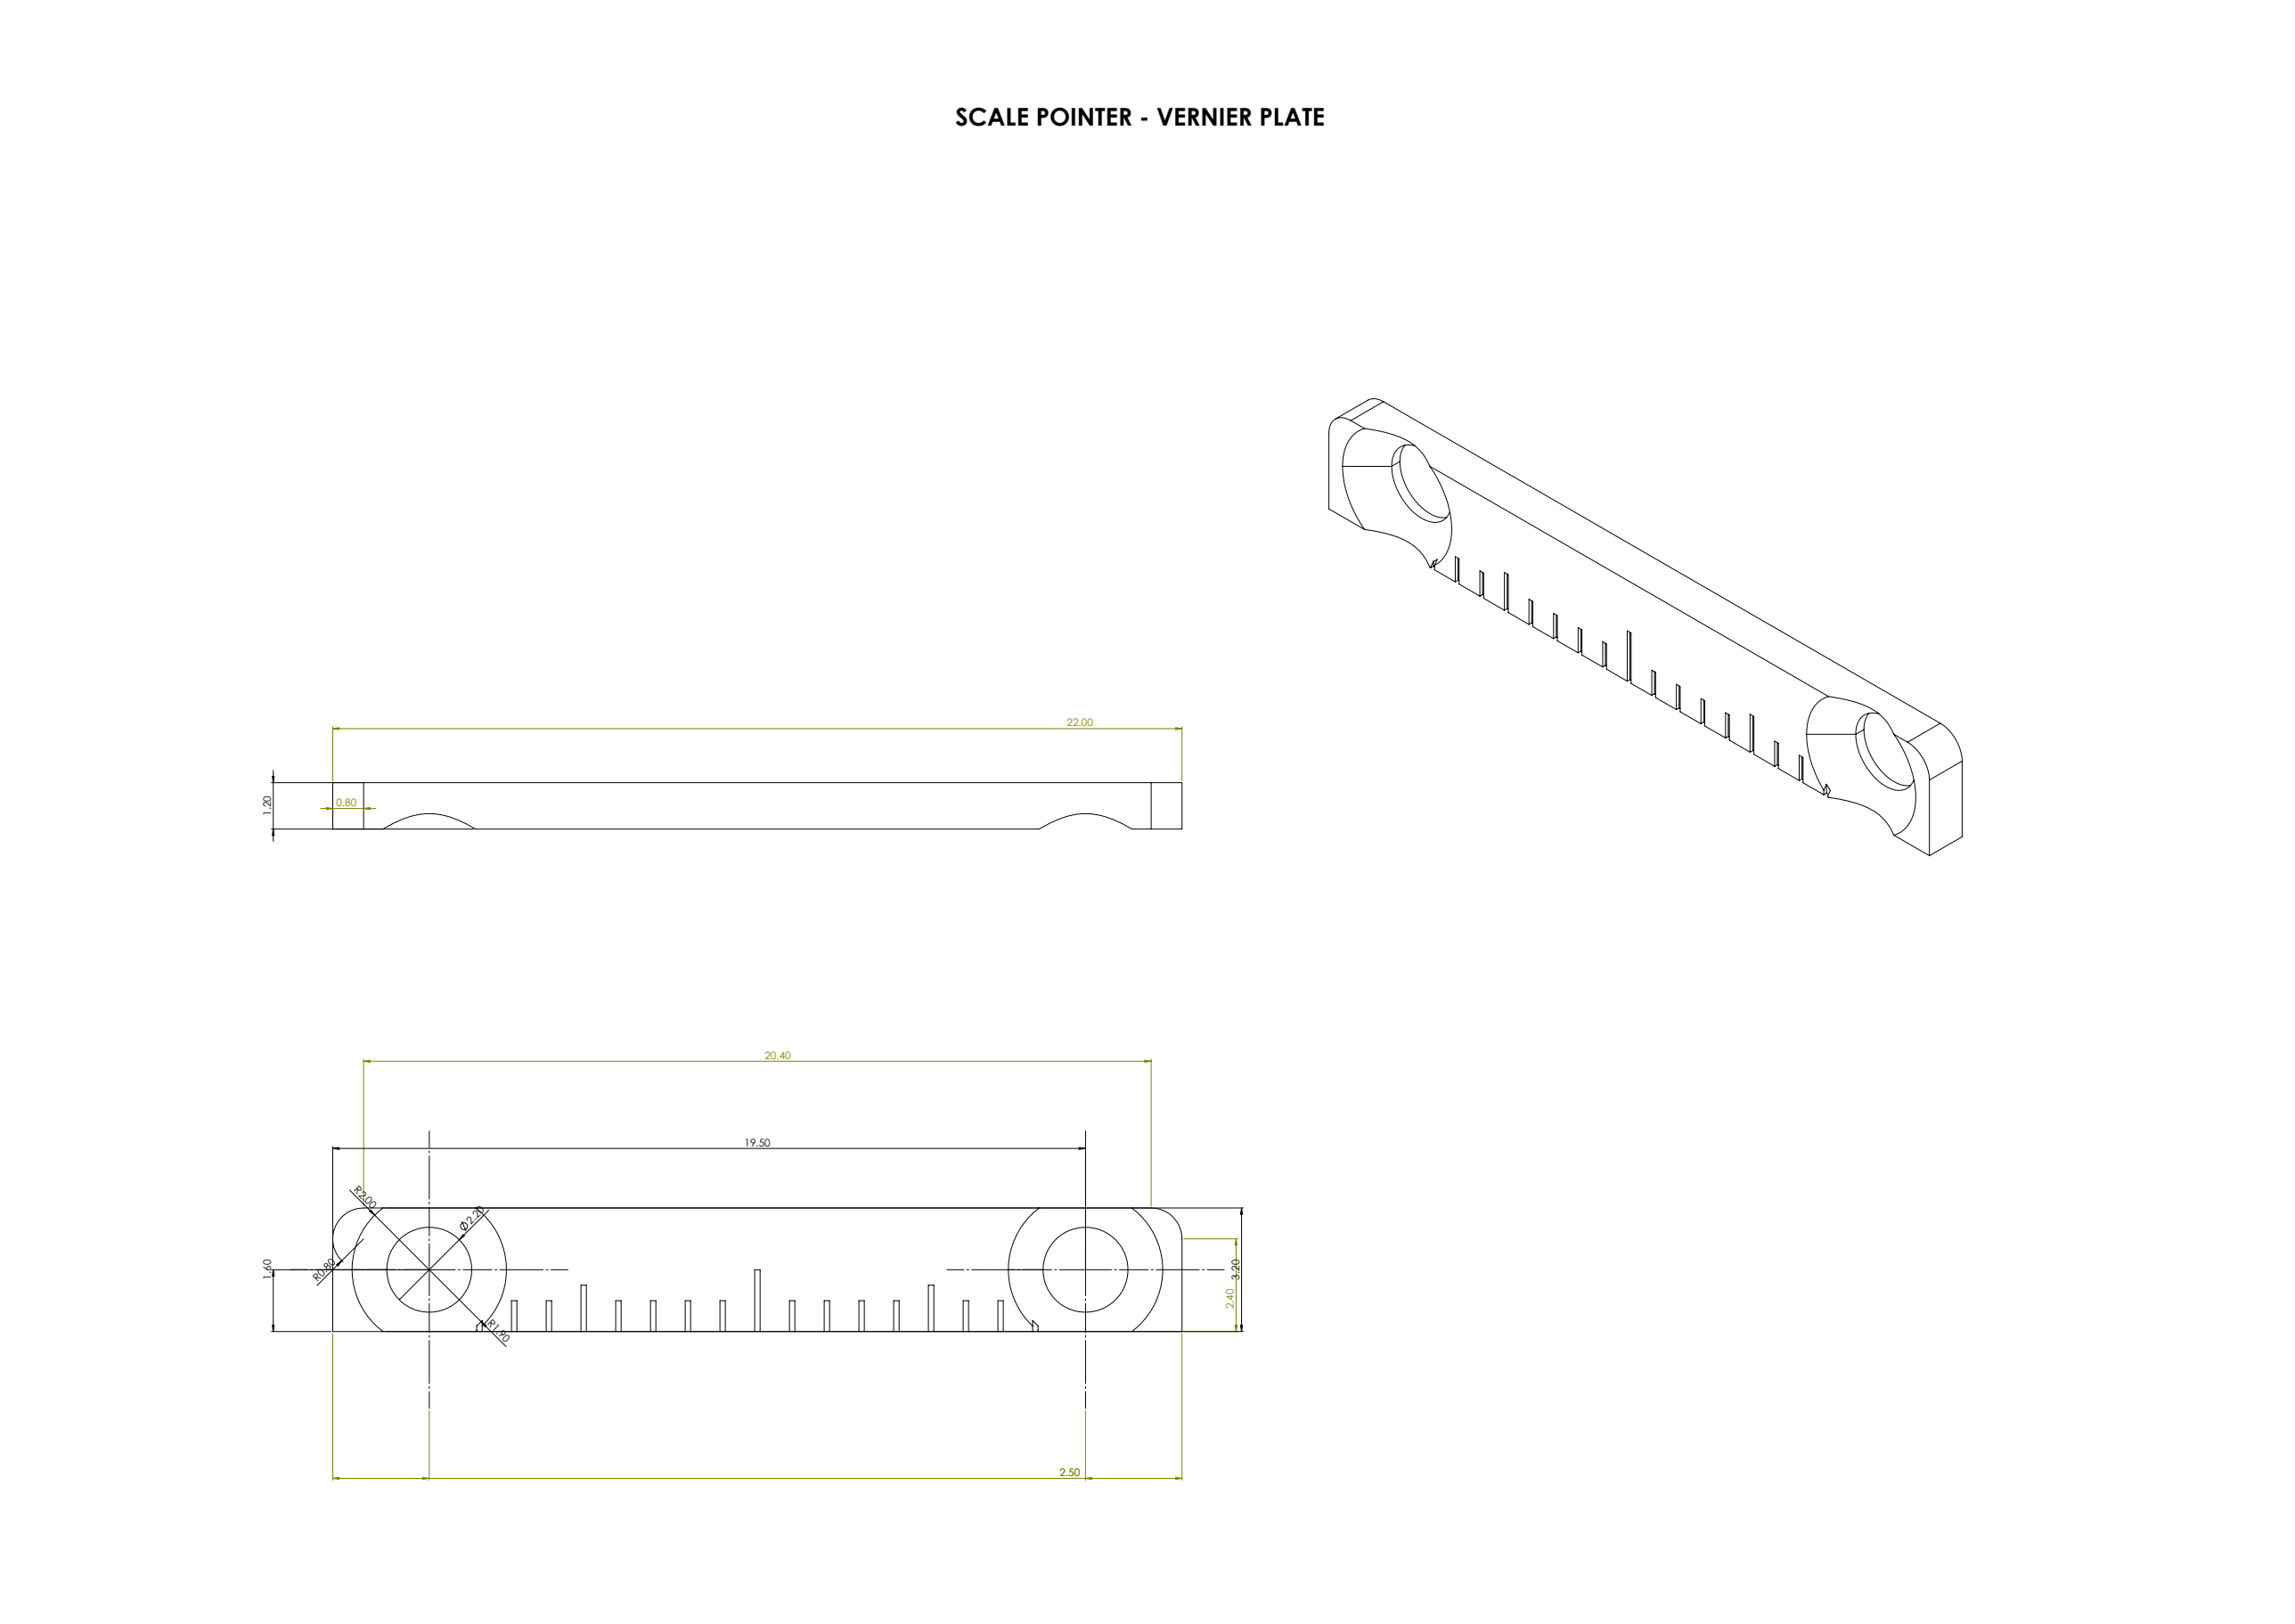
ISO-10303-21;
HEADER;
/* Generated by software containing ST-Developer
 * from STEP Tools, Inc. (www.steptools.com) 
 */

FILE_DESCRIPTION(
/* description */ (''),
/* implementation_level */ '2;1');

FILE_NAME(
/* name */ 'Scale Pointer - Vernier Plate.step',
/* time_stamp */ '2026-10-05T09:57:53+05:00',
/* author */ (''),
/* organization */ (''),
/* preprocessor_version */ 'ST-DEVELOPER v20.2',
/* originating_system */ 'Autodesk Translation Framework v15.15.0.0',
/* authorisation */ '');

FILE_SCHEMA (('AUTOMOTIVE_DESIGN { 1 0 10303 214 3 1 1 }'));
ENDSEC;

DATA;
#10=MECHANICAL_DESIGN_GEOMETRIC_PRESENTATION_REPRESENTATION('',(#560),#113984);
#371=(
BOUNDED_CURVE()
B_SPLINE_CURVE(2,(#102311,#102312,#102313),.UNSPECIFIED.,.F.,.F.)
B_SPLINE_CURVE_WITH_KNOTS((3,3),(0.,0.017254918292991),.UNSPECIFIED.)
CURVE()
GEOMETRIC_REPRESENTATION_ITEM()
RATIONAL_B_SPLINE_CURVE((1.,1.000650607336,1.))
REPRESENTATION_ITEM('')
);
#372=(
BOUNDED_CURVE()
B_SPLINE_CURVE(2,(#102322,#102323,#102324),.UNSPECIFIED.,.F.,.F.)
B_SPLINE_CURVE_WITH_KNOTS((3,3),(0.,0.0163156879194284),.UNSPECIFIED.)
CURVE()
GEOMETRIC_REPRESENTATION_ITEM()
RATIONAL_B_SPLINE_CURVE((1.,1.00054678992472,1.))
REPRESENTATION_ITEM('')
);
#373=(
BOUNDED_CURVE()
B_SPLINE_CURVE(2,(#102497,#102498,#102499),.UNSPECIFIED.,.F.,.F.)
B_SPLINE_CURVE_WITH_KNOTS((3,3),(0.,0.0163156879194291),.UNSPECIFIED.)
CURVE()
GEOMETRIC_REPRESENTATION_ITEM()
RATIONAL_B_SPLINE_CURVE((1.,1.00054678995706,1.))
REPRESENTATION_ITEM('')
);
#374=(
BOUNDED_CURVE()
B_SPLINE_CURVE(2,(#102508,#102509,#102510),.UNSPECIFIED.,.F.,.F.)
B_SPLINE_CURVE_WITH_KNOTS((3,3),(0.,0.0172549182929911),.UNSPECIFIED.)
CURVE()
GEOMETRIC_REPRESENTATION_ITEM()
RATIONAL_B_SPLINE_CURVE((1.,1.0006506073662,1.))
REPRESENTATION_ITEM('')
);
#375=(
BOUNDED_CURVE()
B_SPLINE_CURVE(2,(#102544,#102545,#102546),.UNSPECIFIED.,.F.,.F.)
B_SPLINE_CURVE_WITH_KNOTS((3,3),(0.,0.252982212813465),.UNSPECIFIED.)
CURVE()
GEOMETRIC_REPRESENTATION_ITEM()
RATIONAL_B_SPLINE_CURVE((1.,1.25000000000004,1.))
REPRESENTATION_ITEM('')
);
#376=(
BOUNDED_CURVE()
B_SPLINE_CURVE(2,(#102557,#102558,#102559),.UNSPECIFIED.,.F.,.F.)
B_SPLINE_CURVE_WITH_KNOTS((3,3),(0.,0.252982212813472),.UNSPECIFIED.)
CURVE()
GEOMETRIC_REPRESENTATION_ITEM()
RATIONAL_B_SPLINE_CURVE((1.,1.24999999999997,1.))
REPRESENTATION_ITEM('')
);
#377=(
BOUNDED_CURVE()
B_SPLINE_CURVE(2,(#102574,#102575,#102576),.UNSPECIFIED.,.F.,.F.)
B_SPLINE_CURVE_WITH_KNOTS((3,3),(0.,0.252982212813472),.UNSPECIFIED.)
CURVE()
GEOMETRIC_REPRESENTATION_ITEM()
RATIONAL_B_SPLINE_CURVE((1.,1.24999999999997,1.))
REPRESENTATION_ITEM('')
);
#378=(
BOUNDED_CURVE()
B_SPLINE_CURVE(2,(#102599,#102600,#102601),.UNSPECIFIED.,.F.,.F.)
B_SPLINE_CURVE_WITH_KNOTS((3,3),(0.,0.252982212813465),.UNSPECIFIED.)
CURVE()
GEOMETRIC_REPRESENTATION_ITEM()
RATIONAL_B_SPLINE_CURVE((1.,1.25000000000004,1.))
REPRESENTATION_ITEM('')
);
#524=SHAPE_REPRESENTATION_RELATIONSHIP('SRR','None',#114061,#542);
#542=ADVANCED_BREP_SHAPE_REPRESENTATION('',(#578),#113975);
#560=STYLED_ITEM('',(#114296),#578);
#578=MANIFOLD_SOLID_BREP('Scale Pointer - Vernier Plate',#60401);
#714=CYLINDRICAL_SURFACE('',#63031,1.09999999999999);
#715=CYLINDRICAL_SURFACE('',#63042,1.09999999999999);
#716=CYLINDRICAL_SURFACE('',#63050,0.800000000000001);
#717=CYLINDRICAL_SURFACE('',#63053,0.800000000000001);
#928=CONICAL_SURFACE('',#63034,1.54999999999999,0.785398163397458);
#929=CONICAL_SURFACE('',#63045,1.54999999999999,0.785398163397448);
#1266=CIRCLE('',#62993,1.9);
#1267=CIRCLE('',#63025,1.9);
#1268=CIRCLE('',#63027,2.);
#1269=CIRCLE('',#63029,1.99999999999999);
#1270=CIRCLE('',#63032,1.09999999999999);
#1271=CIRCLE('',#63033,1.09999999999999);
#1272=CIRCLE('',#63035,2.);
#1273=CIRCLE('',#63036,2.);
#1274=CIRCLE('',#63037,2.);
#1275=CIRCLE('',#63039,1.99999999999999);
#1276=CIRCLE('',#63041,0.800000000000001);
#1277=CIRCLE('',#63043,1.09999999999999);
#1278=CIRCLE('',#63044,1.09999999999999);
#1279=CIRCLE('',#63046,1.99999999999999);
#1280=CIRCLE('',#63047,1.99999999999999);
#1281=CIRCLE('',#63049,0.800000000000001);
#1282=CIRCLE('',#63051,0.800000000000001);
#1283=CIRCLE('',#63054,0.800000000000001);
#1849=FACE_BOUND('',#10424,.T.);
#1850=FACE_BOUND('',#10425,.T.);
#3708=PLANE('',#62958);
#3709=PLANE('',#62959);
#3710=PLANE('',#62960);
#3711=PLANE('',#62961);
#3712=PLANE('',#62962);
#3713=PLANE('',#62963);
#3714=PLANE('',#62964);
#3715=PLANE('',#62965);
#3716=PLANE('',#62966);
#3717=PLANE('',#62967);
#3718=PLANE('',#62968);
#3719=PLANE('',#62969);
#3720=PLANE('',#62970);
#3721=PLANE('',#62971);
#3722=PLANE('',#62972);
#3723=PLANE('',#62973);
#3724=PLANE('',#62974);
#3725=PLANE('',#62975);
#3726=PLANE('',#62976);
#3727=PLANE('',#62977);
#3728=PLANE('',#62978);
#3729=PLANE('',#62979);
#3730=PLANE('',#62980);
#3731=PLANE('',#62981);
#3732=PLANE('',#62982);
#3733=PLANE('',#62983);
#3734=PLANE('',#62984);
#3735=PLANE('',#62985);
#3736=PLANE('',#62986);
#3737=PLANE('',#62987);
#3738=PLANE('',#62988);
#3739=PLANE('',#62989);
#3740=PLANE('',#62990);
#3741=PLANE('',#62991);
#3742=PLANE('',#62992);
#3743=PLANE('',#62994);
#3744=PLANE('',#62995);
#3745=PLANE('',#62996);
#3746=PLANE('',#62997);
#3747=PLANE('',#62998);
#3748=PLANE('',#62999);
#3749=PLANE('',#63000);
#3750=PLANE('',#63001);
#3751=PLANE('',#63002);
#3752=PLANE('',#63003);
#3753=PLANE('',#63004);
#3754=PLANE('',#63005);
#3755=PLANE('',#63006);
#3756=PLANE('',#63007);
#3757=PLANE('',#63008);
#3758=PLANE('',#63009);
#3759=PLANE('',#63010);
#3760=PLANE('',#63011);
#3761=PLANE('',#63012);
#3762=PLANE('',#63013);
#3763=PLANE('',#63014);
#3764=PLANE('',#63015);
#3765=PLANE('',#63016);
#3766=PLANE('',#63017);
#3767=PLANE('',#63018);
#3768=PLANE('',#63019);
#3769=PLANE('',#63020);
#3770=PLANE('',#63021);
#3771=PLANE('',#63022);
#3772=PLANE('',#63023);
#3773=PLANE('',#63024);
#3774=PLANE('',#63026);
#3775=PLANE('',#63028);
#3776=PLANE('',#63030);
#3777=PLANE('',#63038);
#3778=PLANE('',#63040);
#3779=PLANE('',#63048);
#3780=PLANE('',#63052);
#3781=PLANE('',#63055);
#3782=PLANE('',#63056);
#3783=PLANE('',#63057);
#6768=FACE_OUTER_BOUND('',#10342,.T.);
#6769=FACE_OUTER_BOUND('',#10343,.T.);
#6770=FACE_OUTER_BOUND('',#10344,.T.);
#6771=FACE_OUTER_BOUND('',#10345,.T.);
#6772=FACE_OUTER_BOUND('',#10346,.T.);
#6773=FACE_OUTER_BOUND('',#10347,.T.);
#6774=FACE_OUTER_BOUND('',#10348,.T.);
#6775=FACE_OUTER_BOUND('',#10349,.T.);
#6776=FACE_OUTER_BOUND('',#10350,.T.);
#6777=FACE_OUTER_BOUND('',#10351,.T.);
#6778=FACE_OUTER_BOUND('',#10352,.T.);
#6779=FACE_OUTER_BOUND('',#10353,.T.);
#6780=FACE_OUTER_BOUND('',#10354,.T.);
#6781=FACE_OUTER_BOUND('',#10355,.T.);
#6782=FACE_OUTER_BOUND('',#10356,.T.);
#6783=FACE_OUTER_BOUND('',#10357,.T.);
#6784=FACE_OUTER_BOUND('',#10358,.T.);
#6785=FACE_OUTER_BOUND('',#10359,.T.);
#6786=FACE_OUTER_BOUND('',#10360,.T.);
#6787=FACE_OUTER_BOUND('',#10361,.T.);
#6788=FACE_OUTER_BOUND('',#10362,.T.);
#6789=FACE_OUTER_BOUND('',#10363,.T.);
#6790=FACE_OUTER_BOUND('',#10364,.T.);
#6791=FACE_OUTER_BOUND('',#10365,.T.);
#6792=FACE_OUTER_BOUND('',#10366,.T.);
#6793=FACE_OUTER_BOUND('',#10367,.T.);
#6794=FACE_OUTER_BOUND('',#10368,.T.);
#6795=FACE_OUTER_BOUND('',#10369,.T.);
#6796=FACE_OUTER_BOUND('',#10370,.T.);
#6797=FACE_OUTER_BOUND('',#10371,.T.);
#6798=FACE_OUTER_BOUND('',#10372,.T.);
#6799=FACE_OUTER_BOUND('',#10373,.T.);
#6800=FACE_OUTER_BOUND('',#10374,.T.);
#6801=FACE_OUTER_BOUND('',#10375,.T.);
#6802=FACE_OUTER_BOUND('',#10376,.T.);
#6803=FACE_OUTER_BOUND('',#10377,.T.);
#6804=FACE_OUTER_BOUND('',#10378,.T.);
#6805=FACE_OUTER_BOUND('',#10379,.T.);
#6806=FACE_OUTER_BOUND('',#10380,.T.);
#6807=FACE_OUTER_BOUND('',#10381,.T.);
#6808=FACE_OUTER_BOUND('',#10382,.T.);
#6809=FACE_OUTER_BOUND('',#10383,.T.);
#6810=FACE_OUTER_BOUND('',#10384,.T.);
#6811=FACE_OUTER_BOUND('',#10385,.T.);
#6812=FACE_OUTER_BOUND('',#10386,.T.);
#6813=FACE_OUTER_BOUND('',#10387,.T.);
#6814=FACE_OUTER_BOUND('',#10388,.T.);
#6815=FACE_OUTER_BOUND('',#10389,.T.);
#6816=FACE_OUTER_BOUND('',#10390,.T.);
#6817=FACE_OUTER_BOUND('',#10391,.T.);
#6818=FACE_OUTER_BOUND('',#10392,.T.);
#6819=FACE_OUTER_BOUND('',#10393,.T.);
#6820=FACE_OUTER_BOUND('',#10394,.T.);
#6821=FACE_OUTER_BOUND('',#10395,.T.);
#6822=FACE_OUTER_BOUND('',#10396,.T.);
#6823=FACE_OUTER_BOUND('',#10397,.T.);
#6824=FACE_OUTER_BOUND('',#10398,.T.);
#6825=FACE_OUTER_BOUND('',#10399,.T.);
#6826=FACE_OUTER_BOUND('',#10400,.T.);
#6827=FACE_OUTER_BOUND('',#10401,.T.);
#6828=FACE_OUTER_BOUND('',#10402,.T.);
#6829=FACE_OUTER_BOUND('',#10403,.T.);
#6830=FACE_OUTER_BOUND('',#10404,.T.);
#6831=FACE_OUTER_BOUND('',#10405,.T.);
#6832=FACE_OUTER_BOUND('',#10406,.T.);
#6833=FACE_OUTER_BOUND('',#10407,.T.);
#6834=FACE_OUTER_BOUND('',#10408,.T.);
#6835=FACE_OUTER_BOUND('',#10409,.T.);
#6836=FACE_OUTER_BOUND('',#10410,.T.);
#6837=FACE_OUTER_BOUND('',#10411,.T.);
#6838=FACE_OUTER_BOUND('',#10412,.T.);
#6839=FACE_OUTER_BOUND('',#10413,.T.);
#6840=FACE_OUTER_BOUND('',#10414,.T.);
#6841=FACE_OUTER_BOUND('',#10415,.T.);
#6842=FACE_OUTER_BOUND('',#10416,.T.);
#6843=FACE_OUTER_BOUND('',#10417,.T.);
#6844=FACE_OUTER_BOUND('',#10418,.T.);
#6845=FACE_OUTER_BOUND('',#10419,.T.);
#6846=FACE_OUTER_BOUND('',#10420,.T.);
#6847=FACE_OUTER_BOUND('',#10421,.T.);
#6848=FACE_OUTER_BOUND('',#10422,.T.);
#6849=FACE_OUTER_BOUND('',#10423,.T.);
#10342=EDGE_LOOP('',(#53603,#53604,#53605,#53606));
#10343=EDGE_LOOP('',(#53607,#53608,#53609,#53610));
#10344=EDGE_LOOP('',(#53611,#53612,#53613,#53614));
#10345=EDGE_LOOP('',(#53615,#53616,#53617,#53618));
#10346=EDGE_LOOP('',(#53619,#53620,#53621,#53622));
#10347=EDGE_LOOP('',(#53623,#53624,#53625,#53626));
#10348=EDGE_LOOP('',(#53627,#53628,#53629,#53630));
#10349=EDGE_LOOP('',(#53631,#53632,#53633,#53634));
#10350=EDGE_LOOP('',(#53635,#53636,#53637,#53638));
#10351=EDGE_LOOP('',(#53639,#53640,#53641,#53642));
#10352=EDGE_LOOP('',(#53643,#53644,#53645,#53646));
#10353=EDGE_LOOP('',(#53647,#53648,#53649,#53650));
#10354=EDGE_LOOP('',(#53651,#53652,#53653,#53654));
#10355=EDGE_LOOP('',(#53655,#53656,#53657,#53658));
#10356=EDGE_LOOP('',(#53659,#53660,#53661,#53662));
#10357=EDGE_LOOP('',(#53663,#53664,#53665,#53666));
#10358=EDGE_LOOP('',(#53667,#53668,#53669,#53670));
#10359=EDGE_LOOP('',(#53671,#53672,#53673,#53674));
#10360=EDGE_LOOP('',(#53675,#53676,#53677,#53678));
#10361=EDGE_LOOP('',(#53679,#53680,#53681,#53682));
#10362=EDGE_LOOP('',(#53683,#53684,#53685,#53686));
#10363=EDGE_LOOP('',(#53687,#53688,#53689,#53690));
#10364=EDGE_LOOP('',(#53691,#53692,#53693,#53694));
#10365=EDGE_LOOP('',(#53695,#53696,#53697,#53698));
#10366=EDGE_LOOP('',(#53699,#53700,#53701,#53702));
#10367=EDGE_LOOP('',(#53703,#53704,#53705,#53706));
#10368=EDGE_LOOP('',(#53707,#53708,#53709,#53710));
#10369=EDGE_LOOP('',(#53711,#53712,#53713,#53714));
#10370=EDGE_LOOP('',(#53715,#53716,#53717,#53718));
#10371=EDGE_LOOP('',(#53719,#53720,#53721,#53722));
#10372=EDGE_LOOP('',(#53723,#53724,#53725,#53726));
#10373=EDGE_LOOP('',(#53727,#53728,#53729,#53730));
#10374=EDGE_LOOP('',(#53731,#53732,#53733,#53734));
#10375=EDGE_LOOP('',(#53735,#53736,#53737,#53738));
#10376=EDGE_LOOP('',(#53739,#53740,#53741,#53742));
#10377=EDGE_LOOP('',(#53743,#53744,#53745,#53746));
#10378=EDGE_LOOP('',(#53747,#53748,#53749,#53750));
#10379=EDGE_LOOP('',(#53751,#53752,#53753,#53754));
#10380=EDGE_LOOP('',(#53755,#53756,#53757,#53758));
#10381=EDGE_LOOP('',(#53759,#53760,#53761,#53762));
#10382=EDGE_LOOP('',(#53763,#53764,#53765,#53766));
#10383=EDGE_LOOP('',(#53767,#53768,#53769,#53770));
#10384=EDGE_LOOP('',(#53771,#53772,#53773,#53774));
#10385=EDGE_LOOP('',(#53775,#53776,#53777,#53778));
#10386=EDGE_LOOP('',(#53779,#53780,#53781,#53782));
#10387=EDGE_LOOP('',(#53783,#53784,#53785,#53786));
#10388=EDGE_LOOP('',(#53787,#53788,#53789,#53790));
#10389=EDGE_LOOP('',(#53791,#53792,#53793,#53794));
#10390=EDGE_LOOP('',(#53795,#53796,#53797,#53798));
#10391=EDGE_LOOP('',(#53799,#53800,#53801,#53802));
#10392=EDGE_LOOP('',(#53803,#53804,#53805,#53806));
#10393=EDGE_LOOP('',(#53807,#53808,#53809,#53810));
#10394=EDGE_LOOP('',(#53811,#53812,#53813,#53814));
#10395=EDGE_LOOP('',(#53815,#53816,#53817,#53818));
#10396=EDGE_LOOP('',(#53819,#53820,#53821,#53822));
#10397=EDGE_LOOP('',(#53823,#53824,#53825,#53826));
#10398=EDGE_LOOP('',(#53827,#53828,#53829,#53830));
#10399=EDGE_LOOP('',(#53831,#53832,#53833,#53834));
#10400=EDGE_LOOP('',(#53835,#53836,#53837,#53838));
#10401=EDGE_LOOP('',(#53839,#53840,#53841,#53842));
#10402=EDGE_LOOP('',(#53843,#53844,#53845,#53846));
#10403=EDGE_LOOP('',(#53847,#53848,#53849,#53850));
#10404=EDGE_LOOP('',(#53851,#53852,#53853,#53854));
#10405=EDGE_LOOP('',(#53855,#53856,#53857,#53858));
#10406=EDGE_LOOP('',(#53859,#53860,#53861,#53862));
#10407=EDGE_LOOP('',(#53863,#53864,#53865,#53866));
#10408=EDGE_LOOP('',(#53867,#53868,#53869));
#10409=EDGE_LOOP('',(#53870,#53871,#53872));
#10410=EDGE_LOOP('',(#53873,#53874,#53875,#53876,#53877,#53878,#53879,#53880,
#53881,#53882,#53883,#53884,#53885,#53886,#53887,#53888,#53889,#53890,#53891,
#53892,#53893,#53894,#53895,#53896,#53897,#53898,#53899,#53900,#53901,#53902,
#53903,#53904,#53905,#53906,#53907,#53908,#53909,#53910,#53911,#53912,#53913,
#53914,#53915,#53916,#53917,#53918,#53919,#53920,#53921,#53922,#53923,#53924,
#53925,#53926,#53927,#53928,#53929,#53930,#53931,#53932,#53933,#53934,#53935,
#53936,#53937,#53938,#53939,#53940,#53941,#53942,#53943,#53944,#53945,#53946,
#53947,#53948));
#10411=EDGE_LOOP('',(#53949,#53950,#53951,#53952));
#10412=EDGE_LOOP('',(#53953,#53954,#53955,#53956,#53957,#53958,#53959,#53960,
#53961,#53962,#53963,#53964));
#10413=EDGE_LOOP('',(#53965,#53966,#53967,#53968,#53969,#53970,#53971,#53972,
#53973,#53974,#53975,#53976,#53977,#53978,#53979,#53980,#53981,#53982,#53983,
#53984,#53985,#53986,#53987,#53988,#53989,#53990,#53991,#53992,#53993,#53994,
#53995,#53996,#53997,#53998,#53999,#54000,#54001,#54002,#54003,#54004,#54005,
#54006,#54007,#54008,#54009,#54010,#54011,#54012,#54013,#54014,#54015,#54016,
#54017,#54018,#54019,#54020,#54021,#54022,#54023,#54024,#54025,#54026,#54027,
#54028,#54029,#54030,#54031));
#10414=EDGE_LOOP('',(#54032,#54033,#54034,#54035,#54036));
#10415=EDGE_LOOP('',(#54037,#54038,#54039,#54040));
#10416=EDGE_LOOP('',(#54041,#54042,#54043,#54044,#54045,#54046,#54047,#54048,
#54049,#54050,#54051,#54052));
#10417=EDGE_LOOP('',(#54053,#54054,#54055,#54056,#54057,#54058));
#10418=EDGE_LOOP('',(#54059,#54060,#54061,#54062));
#10419=EDGE_LOOP('',(#54063,#54064,#54065,#54066,#54067,#54068,#54069,#54070));
#10420=EDGE_LOOP('',(#54071,#54072,#54073,#54074));
#10421=EDGE_LOOP('',(#54075,#54076,#54077,#54078));
#10422=EDGE_LOOP('',(#54079,#54080,#54081,#54082));
#10423=EDGE_LOOP('',(#54083,#54084,#54085,#54086,#54087,#54088));
#10424=EDGE_LOOP('',(#54089));
#10425=EDGE_LOOP('',(#54090));
#16198=LINE('',#102127,#22232);
#16199=LINE('',#102129,#22233);
#16200=LINE('',#102131,#22234);
#16201=LINE('',#102132,#22235);
#16202=LINE('',#102135,#22236);
#16203=LINE('',#102137,#22237);
#16204=LINE('',#102138,#22238);
#16205=LINE('',#102141,#22239);
#16206=LINE('',#102142,#22240);
#16207=LINE('',#102145,#22241);
#16208=LINE('',#102146,#22242);
#16209=LINE('',#102150,#22243);
#16210=LINE('',#102152,#22244);
#16211=LINE('',#102154,#22245);
#16212=LINE('',#102155,#22246);
#16213=LINE('',#102158,#22247);
#16214=LINE('',#102160,#22248);
#16215=LINE('',#102161,#22249);
#16216=LINE('',#102164,#22250);
#16217=LINE('',#102165,#22251);
#16218=LINE('',#102168,#22252);
#16219=LINE('',#102169,#22253);
#16220=LINE('',#102173,#22254);
#16221=LINE('',#102175,#22255);
#16222=LINE('',#102177,#22256);
#16223=LINE('',#102178,#22257);
#16224=LINE('',#102181,#22258);
#16225=LINE('',#102183,#22259);
#16226=LINE('',#102184,#22260);
#16227=LINE('',#102187,#22261);
#16228=LINE('',#102188,#22262);
#16229=LINE('',#102191,#22263);
#16230=LINE('',#102192,#22264);
#16231=LINE('',#102196,#22265);
#16232=LINE('',#102198,#22266);
#16233=LINE('',#102200,#22267);
#16234=LINE('',#102201,#22268);
#16235=LINE('',#102204,#22269);
#16236=LINE('',#102206,#22270);
#16237=LINE('',#102207,#22271);
#16238=LINE('',#102210,#22272);
#16239=LINE('',#102211,#22273);
#16240=LINE('',#102214,#22274);
#16241=LINE('',#102215,#22275);
#16242=LINE('',#102219,#22276);
#16243=LINE('',#102221,#22277);
#16244=LINE('',#102223,#22278);
#16245=LINE('',#102224,#22279);
#16246=LINE('',#102227,#22280);
#16247=LINE('',#102229,#22281);
#16248=LINE('',#102230,#22282);
#16249=LINE('',#102233,#22283);
#16250=LINE('',#102234,#22284);
#16251=LINE('',#102237,#22285);
#16252=LINE('',#102238,#22286);
#16253=LINE('',#102242,#22287);
#16254=LINE('',#102244,#22288);
#16255=LINE('',#102246,#22289);
#16256=LINE('',#102247,#22290);
#16257=LINE('',#102250,#22291);
#16258=LINE('',#102252,#22292);
#16259=LINE('',#102253,#22293);
#16260=LINE('',#102256,#22294);
#16261=LINE('',#102257,#22295);
#16262=LINE('',#102260,#22296);
#16263=LINE('',#102261,#22297);
#16264=LINE('',#102265,#22298);
#16265=LINE('',#102267,#22299);
#16266=LINE('',#102269,#22300);
#16267=LINE('',#102270,#22301);
#16268=LINE('',#102273,#22302);
#16269=LINE('',#102275,#22303);
#16270=LINE('',#102276,#22304);
#16271=LINE('',#102279,#22305);
#16272=LINE('',#102280,#22306);
#16273=LINE('',#102283,#22307);
#16274=LINE('',#102284,#22308);
#16275=LINE('',#102288,#22309);
#16276=LINE('',#102290,#22310);
#16277=LINE('',#102292,#22311);
#16278=LINE('',#102293,#22312);
#16279=LINE('',#102296,#22313);
#16280=LINE('',#102298,#22314);
#16281=LINE('',#102299,#22315);
#16282=LINE('',#102302,#22316);
#16283=LINE('',#102303,#22317);
#16284=LINE('',#102306,#22318);
#16285=LINE('',#102307,#22319);
#16286=LINE('',#102315,#22320);
#16287=LINE('',#102317,#22321);
#16288=LINE('',#102318,#22322);
#16289=LINE('',#102326,#22323);
#16290=LINE('',#102328,#22324);
#16291=LINE('',#102329,#22325);
#16292=LINE('',#102332,#22326);
#16293=LINE('',#102336,#22327);
#16294=LINE('',#102338,#22328);
#16295=LINE('',#102340,#22329);
#16296=LINE('',#102341,#22330);
#16297=LINE('',#102344,#22331);
#16298=LINE('',#102346,#22332);
#16299=LINE('',#102347,#22333);
#16300=LINE('',#102350,#22334);
#16301=LINE('',#102351,#22335);
#16302=LINE('',#102354,#22336);
#16303=LINE('',#102355,#22337);
#16304=LINE('',#102359,#22338);
#16305=LINE('',#102361,#22339);
#16306=LINE('',#102363,#22340);
#16307=LINE('',#102364,#22341);
#16308=LINE('',#102367,#22342);
#16309=LINE('',#102369,#22343);
#16310=LINE('',#102370,#22344);
#16311=LINE('',#102373,#22345);
#16312=LINE('',#102374,#22346);
#16313=LINE('',#102377,#22347);
#16314=LINE('',#102378,#22348);
#16315=LINE('',#102382,#22349);
#16316=LINE('',#102384,#22350);
#16317=LINE('',#102386,#22351);
#16318=LINE('',#102387,#22352);
#16319=LINE('',#102390,#22353);
#16320=LINE('',#102392,#22354);
#16321=LINE('',#102393,#22355);
#16322=LINE('',#102396,#22356);
#16323=LINE('',#102397,#22357);
#16324=LINE('',#102400,#22358);
#16325=LINE('',#102401,#22359);
#16326=LINE('',#102405,#22360);
#16327=LINE('',#102407,#22361);
#16328=LINE('',#102409,#22362);
#16329=LINE('',#102410,#22363);
#16330=LINE('',#102413,#22364);
#16331=LINE('',#102415,#22365);
#16332=LINE('',#102416,#22366);
#16333=LINE('',#102419,#22367);
#16334=LINE('',#102420,#22368);
#16335=LINE('',#102423,#22369);
#16336=LINE('',#102424,#22370);
#16337=LINE('',#102428,#22371);
#16338=LINE('',#102430,#22372);
#16339=LINE('',#102432,#22373);
#16340=LINE('',#102433,#22374);
#16341=LINE('',#102436,#22375);
#16342=LINE('',#102438,#22376);
#16343=LINE('',#102439,#22377);
#16344=LINE('',#102442,#22378);
#16345=LINE('',#102443,#22379);
#16346=LINE('',#102446,#22380);
#16347=LINE('',#102447,#22381);
#16348=LINE('',#102451,#22382);
#16349=LINE('',#102453,#22383);
#16350=LINE('',#102455,#22384);
#16351=LINE('',#102456,#22385);
#16352=LINE('',#102459,#22386);
#16353=LINE('',#102461,#22387);
#16354=LINE('',#102462,#22388);
#16355=LINE('',#102465,#22389);
#16356=LINE('',#102466,#22390);
#16357=LINE('',#102469,#22391);
#16358=LINE('',#102470,#22392);
#16359=LINE('',#102474,#22393);
#16360=LINE('',#102476,#22394);
#16361=LINE('',#102478,#22395);
#16362=LINE('',#102479,#22396);
#16363=LINE('',#102482,#22397);
#16364=LINE('',#102484,#22398);
#16365=LINE('',#102485,#22399);
#16366=LINE('',#102488,#22400);
#16367=LINE('',#102489,#22401);
#16368=LINE('',#102492,#22402);
#16369=LINE('',#102493,#22403);
#16370=LINE('',#102501,#22404);
#16371=LINE('',#102503,#22405);
#16372=LINE('',#102504,#22406);
#16373=LINE('',#102512,#22407);
#16374=LINE('',#102514,#22408);
#16375=LINE('',#102515,#22409);
#16376=LINE('',#102518,#22410);
#16377=LINE('',#102521,#22411);
#16378=LINE('',#102526,#22412);
#16379=LINE('',#102528,#22413);
#16380=LINE('',#102529,#22414);
#16381=LINE('',#102530,#22415);
#16382=LINE('',#102531,#22416);
#16383=LINE('',#102532,#22417);
#16384=LINE('',#102533,#22418);
#16385=LINE('',#102534,#22419);
#16386=LINE('',#102535,#22420);
#16387=LINE('',#102536,#22421);
#16388=LINE('',#102537,#22422);
#16389=LINE('',#102538,#22423);
#16390=LINE('',#102539,#22424);
#16391=LINE('',#102540,#22425);
#16392=LINE('',#102541,#22426);
#16393=LINE('',#102542,#22427);
#16394=LINE('',#102548,#22428);
#16395=LINE('',#102550,#22429);
#16396=LINE('',#102552,#22430);
#16397=LINE('',#102554,#22431);
#16398=LINE('',#102556,#22432);
#16399=LINE('',#102560,#22433);
#16400=LINE('',#102565,#22434);
#16401=LINE('',#102569,#22435);
#16402=LINE('',#102580,#22436);
#16403=LINE('',#102584,#22437);
#16404=LINE('',#102587,#22438);
#16405=LINE('',#102592,#22439);
#16406=LINE('',#102596,#22440);
#16407=LINE('',#102605,#22441);
#16408=LINE('',#102608,#22442);
#16409=LINE('',#102613,#22443);
#16410=LINE('',#102614,#22444);
#16411=LINE('',#102617,#22445);
#16412=LINE('',#102618,#22446);
#16413=LINE('',#102622,#22447);
#16414=LINE('',#102624,#22448);
#16415=LINE('',#102626,#22449);
#22232=VECTOR('',#73798,10.);
#22233=VECTOR('',#73799,10.);
#22234=VECTOR('',#73800,10.);
#22235=VECTOR('',#73801,10.);
#22236=VECTOR('',#73804,10.);
#22237=VECTOR('',#73805,10.);
#22238=VECTOR('',#73806,10.);
#22239=VECTOR('',#73809,10.);
#22240=VECTOR('',#73810,10.);
#22241=VECTOR('',#73813,10.);
#22242=VECTOR('',#73814,10.);
#22243=VECTOR('',#73817,10.);
#22244=VECTOR('',#73818,10.);
#22245=VECTOR('',#73819,10.);
#22246=VECTOR('',#73820,10.);
#22247=VECTOR('',#73823,10.);
#22248=VECTOR('',#73824,10.);
#22249=VECTOR('',#73825,10.);
#22250=VECTOR('',#73828,10.);
#22251=VECTOR('',#73829,10.);
#22252=VECTOR('',#73832,10.);
#22253=VECTOR('',#73833,10.);
#22254=VECTOR('',#73836,10.);
#22255=VECTOR('',#73837,10.);
#22256=VECTOR('',#73838,10.);
#22257=VECTOR('',#73839,10.);
#22258=VECTOR('',#73842,10.);
#22259=VECTOR('',#73843,10.);
#22260=VECTOR('',#73844,10.);
#22261=VECTOR('',#73847,10.);
#22262=VECTOR('',#73848,10.);
#22263=VECTOR('',#73851,10.);
#22264=VECTOR('',#73852,10.);
#22265=VECTOR('',#73855,10.);
#22266=VECTOR('',#73856,10.);
#22267=VECTOR('',#73857,10.);
#22268=VECTOR('',#73858,10.);
#22269=VECTOR('',#73861,10.);
#22270=VECTOR('',#73862,10.);
#22271=VECTOR('',#73863,10.);
#22272=VECTOR('',#73866,10.);
#22273=VECTOR('',#73867,10.);
#22274=VECTOR('',#73870,10.);
#22275=VECTOR('',#73871,10.);
#22276=VECTOR('',#73874,10.);
#22277=VECTOR('',#73875,10.);
#22278=VECTOR('',#73876,10.);
#22279=VECTOR('',#73877,10.);
#22280=VECTOR('',#73880,10.);
#22281=VECTOR('',#73881,10.);
#22282=VECTOR('',#73882,10.);
#22283=VECTOR('',#73885,10.);
#22284=VECTOR('',#73886,10.);
#22285=VECTOR('',#73889,10.);
#22286=VECTOR('',#73890,10.);
#22287=VECTOR('',#73893,10.);
#22288=VECTOR('',#73894,10.);
#22289=VECTOR('',#73895,10.);
#22290=VECTOR('',#73896,10.);
#22291=VECTOR('',#73899,10.);
#22292=VECTOR('',#73900,10.);
#22293=VECTOR('',#73901,10.);
#22294=VECTOR('',#73904,10.);
#22295=VECTOR('',#73905,10.);
#22296=VECTOR('',#73908,10.);
#22297=VECTOR('',#73909,10.);
#22298=VECTOR('',#73912,10.);
#22299=VECTOR('',#73913,10.);
#22300=VECTOR('',#73914,10.);
#22301=VECTOR('',#73915,10.);
#22302=VECTOR('',#73918,10.);
#22303=VECTOR('',#73919,10.);
#22304=VECTOR('',#73920,10.);
#22305=VECTOR('',#73923,10.);
#22306=VECTOR('',#73924,10.);
#22307=VECTOR('',#73927,10.);
#22308=VECTOR('',#73928,10.);
#22309=VECTOR('',#73931,10.);
#22310=VECTOR('',#73932,10.);
#22311=VECTOR('',#73933,10.);
#22312=VECTOR('',#73934,10.);
#22313=VECTOR('',#73937,10.);
#22314=VECTOR('',#73938,10.);
#22315=VECTOR('',#73939,10.);
#22316=VECTOR('',#73942,10.);
#22317=VECTOR('',#73943,10.);
#22318=VECTOR('',#73946,10.);
#22319=VECTOR('',#73947,10.);
#22320=VECTOR('',#73950,10.);
#22321=VECTOR('',#73951,10.);
#22322=VECTOR('',#73952,10.);
#22323=VECTOR('',#73955,10.);
#22324=VECTOR('',#73956,10.);
#22325=VECTOR('',#73957,10.);
#22326=VECTOR('',#73962,10.);
#22327=VECTOR('',#73965,10.);
#22328=VECTOR('',#73966,10.);
#22329=VECTOR('',#73967,10.);
#22330=VECTOR('',#73968,10.);
#22331=VECTOR('',#73971,10.);
#22332=VECTOR('',#73972,10.);
#22333=VECTOR('',#73973,10.);
#22334=VECTOR('',#73976,10.);
#22335=VECTOR('',#73977,10.);
#22336=VECTOR('',#73980,10.);
#22337=VECTOR('',#73981,10.);
#22338=VECTOR('',#73984,10.);
#22339=VECTOR('',#73985,10.);
#22340=VECTOR('',#73986,10.);
#22341=VECTOR('',#73987,10.);
#22342=VECTOR('',#73990,10.);
#22343=VECTOR('',#73991,10.);
#22344=VECTOR('',#73992,10.);
#22345=VECTOR('',#73995,10.);
#22346=VECTOR('',#73996,10.);
#22347=VECTOR('',#73999,10.);
#22348=VECTOR('',#74000,10.);
#22349=VECTOR('',#74003,10.);
#22350=VECTOR('',#74004,10.);
#22351=VECTOR('',#74005,10.);
#22352=VECTOR('',#74006,10.);
#22353=VECTOR('',#74009,10.);
#22354=VECTOR('',#74010,10.);
#22355=VECTOR('',#74011,10.);
#22356=VECTOR('',#74014,10.);
#22357=VECTOR('',#74015,10.);
#22358=VECTOR('',#74018,10.);
#22359=VECTOR('',#74019,10.);
#22360=VECTOR('',#74022,10.);
#22361=VECTOR('',#74023,10.);
#22362=VECTOR('',#74024,10.);
#22363=VECTOR('',#74025,10.);
#22364=VECTOR('',#74028,10.);
#22365=VECTOR('',#74029,10.);
#22366=VECTOR('',#74030,10.);
#22367=VECTOR('',#74033,10.);
#22368=VECTOR('',#74034,10.);
#22369=VECTOR('',#74037,10.);
#22370=VECTOR('',#74038,10.);
#22371=VECTOR('',#74041,10.);
#22372=VECTOR('',#74042,10.);
#22373=VECTOR('',#74043,10.);
#22374=VECTOR('',#74044,10.);
#22375=VECTOR('',#74047,10.);
#22376=VECTOR('',#74048,10.);
#22377=VECTOR('',#74049,10.);
#22378=VECTOR('',#74052,10.);
#22379=VECTOR('',#74053,10.);
#22380=VECTOR('',#74056,10.);
#22381=VECTOR('',#74057,10.);
#22382=VECTOR('',#74060,10.);
#22383=VECTOR('',#74061,10.);
#22384=VECTOR('',#74062,10.);
#22385=VECTOR('',#74063,10.);
#22386=VECTOR('',#74066,10.);
#22387=VECTOR('',#74067,10.);
#22388=VECTOR('',#74068,10.);
#22389=VECTOR('',#74071,10.);
#22390=VECTOR('',#74072,10.);
#22391=VECTOR('',#74075,10.);
#22392=VECTOR('',#74076,10.);
#22393=VECTOR('',#74079,10.);
#22394=VECTOR('',#74080,10.);
#22395=VECTOR('',#74081,10.);
#22396=VECTOR('',#74082,10.);
#22397=VECTOR('',#74085,10.);
#22398=VECTOR('',#74086,10.);
#22399=VECTOR('',#74087,10.);
#22400=VECTOR('',#74090,10.);
#22401=VECTOR('',#74091,10.);
#22402=VECTOR('',#74094,10.);
#22403=VECTOR('',#74095,10.);
#22404=VECTOR('',#74098,10.);
#22405=VECTOR('',#74099,10.);
#22406=VECTOR('',#74100,10.);
#22407=VECTOR('',#74103,10.);
#22408=VECTOR('',#74104,10.);
#22409=VECTOR('',#74105,10.);
#22410=VECTOR('',#74110,10.);
#22411=VECTOR('',#74113,10.);
#22412=VECTOR('',#74120,10.);
#22413=VECTOR('',#74123,10.);
#22414=VECTOR('',#74124,10.);
#22415=VECTOR('',#74125,10.);
#22416=VECTOR('',#74126,10.);
#22417=VECTOR('',#74127,10.);
#22418=VECTOR('',#74128,10.);
#22419=VECTOR('',#74129,10.);
#22420=VECTOR('',#74130,10.);
#22421=VECTOR('',#74131,10.);
#22422=VECTOR('',#74132,10.);
#22423=VECTOR('',#74133,10.);
#22424=VECTOR('',#74134,10.);
#22425=VECTOR('',#74135,10.);
#22426=VECTOR('',#74136,10.);
#22427=VECTOR('',#74137,10.);
#22428=VECTOR('',#74138,10.);
#22429=VECTOR('',#74139,10.);
#22430=VECTOR('',#74140,10.);
#22431=VECTOR('',#74141,10.);
#22432=VECTOR('',#74142,10.);
#22433=VECTOR('',#74143,10.);
#22434=VECTOR('',#74148,1.09999999999999);
#22435=VECTOR('',#74153,1.54999999999999);
#22436=VECTOR('',#74162,10.);
#22437=VECTOR('',#74167,10.);
#22438=VECTOR('',#74170,10.);
#22439=VECTOR('',#74175,1.09999999999999);
#22440=VECTOR('',#74180,1.54999999999999);
#22441=VECTOR('',#74187,10.);
#22442=VECTOR('',#74190,10.);
#22443=VECTOR('',#74195,10.);
#22444=VECTOR('',#74196,10.);
#22445=VECTOR('',#74199,10.);
#22446=VECTOR('',#74200,10.);
#22447=VECTOR('',#74205,10.);
#22448=VECTOR('',#74208,10.);
#22449=VECTOR('',#74211,10.);
#29447=VERTEX_POINT('',#102125);
#29448=VERTEX_POINT('',#102126);
#29449=VERTEX_POINT('',#102128);
#29450=VERTEX_POINT('',#102130);
#29451=VERTEX_POINT('',#102134);
#29452=VERTEX_POINT('',#102136);
#29453=VERTEX_POINT('',#102140);
#29454=VERTEX_POINT('',#102144);
#29455=VERTEX_POINT('',#102148);
#29456=VERTEX_POINT('',#102149);
#29457=VERTEX_POINT('',#102151);
#29458=VERTEX_POINT('',#102153);
#29459=VERTEX_POINT('',#102157);
#29460=VERTEX_POINT('',#102159);
#29461=VERTEX_POINT('',#102163);
#29462=VERTEX_POINT('',#102167);
#29463=VERTEX_POINT('',#102171);
#29464=VERTEX_POINT('',#102172);
#29465=VERTEX_POINT('',#102174);
#29466=VERTEX_POINT('',#102176);
#29467=VERTEX_POINT('',#102180);
#29468=VERTEX_POINT('',#102182);
#29469=VERTEX_POINT('',#102186);
#29470=VERTEX_POINT('',#102190);
#29471=VERTEX_POINT('',#102194);
#29472=VERTEX_POINT('',#102195);
#29473=VERTEX_POINT('',#102197);
#29474=VERTEX_POINT('',#102199);
#29475=VERTEX_POINT('',#102203);
#29476=VERTEX_POINT('',#102205);
#29477=VERTEX_POINT('',#102209);
#29478=VERTEX_POINT('',#102213);
#29479=VERTEX_POINT('',#102217);
#29480=VERTEX_POINT('',#102218);
#29481=VERTEX_POINT('',#102220);
#29482=VERTEX_POINT('',#102222);
#29483=VERTEX_POINT('',#102226);
#29484=VERTEX_POINT('',#102228);
#29485=VERTEX_POINT('',#102232);
#29486=VERTEX_POINT('',#102236);
#29487=VERTEX_POINT('',#102240);
#29488=VERTEX_POINT('',#102241);
#29489=VERTEX_POINT('',#102243);
#29490=VERTEX_POINT('',#102245);
#29491=VERTEX_POINT('',#102249);
#29492=VERTEX_POINT('',#102251);
#29493=VERTEX_POINT('',#102255);
#29494=VERTEX_POINT('',#102259);
#29495=VERTEX_POINT('',#102263);
#29496=VERTEX_POINT('',#102264);
#29497=VERTEX_POINT('',#102266);
#29498=VERTEX_POINT('',#102268);
#29499=VERTEX_POINT('',#102272);
#29500=VERTEX_POINT('',#102274);
#29501=VERTEX_POINT('',#102278);
#29502=VERTEX_POINT('',#102282);
#29503=VERTEX_POINT('',#102286);
#29504=VERTEX_POINT('',#102287);
#29505=VERTEX_POINT('',#102289);
#29506=VERTEX_POINT('',#102291);
#29507=VERTEX_POINT('',#102295);
#29508=VERTEX_POINT('',#102297);
#29509=VERTEX_POINT('',#102301);
#29510=VERTEX_POINT('',#102305);
#29511=VERTEX_POINT('',#102309);
#29512=VERTEX_POINT('',#102310);
#29513=VERTEX_POINT('',#102314);
#29514=VERTEX_POINT('',#102316);
#29515=VERTEX_POINT('',#102320);
#29516=VERTEX_POINT('',#102321);
#29517=VERTEX_POINT('',#102325);
#29518=VERTEX_POINT('',#102327);
#29519=VERTEX_POINT('',#102334);
#29520=VERTEX_POINT('',#102335);
#29521=VERTEX_POINT('',#102337);
#29522=VERTEX_POINT('',#102339);
#29523=VERTEX_POINT('',#102343);
#29524=VERTEX_POINT('',#102345);
#29525=VERTEX_POINT('',#102349);
#29526=VERTEX_POINT('',#102353);
#29527=VERTEX_POINT('',#102357);
#29528=VERTEX_POINT('',#102358);
#29529=VERTEX_POINT('',#102360);
#29530=VERTEX_POINT('',#102362);
#29531=VERTEX_POINT('',#102366);
#29532=VERTEX_POINT('',#102368);
#29533=VERTEX_POINT('',#102372);
#29534=VERTEX_POINT('',#102376);
#29535=VERTEX_POINT('',#102380);
#29536=VERTEX_POINT('',#102381);
#29537=VERTEX_POINT('',#102383);
#29538=VERTEX_POINT('',#102385);
#29539=VERTEX_POINT('',#102389);
#29540=VERTEX_POINT('',#102391);
#29541=VERTEX_POINT('',#102395);
#29542=VERTEX_POINT('',#102399);
#29543=VERTEX_POINT('',#102403);
#29544=VERTEX_POINT('',#102404);
#29545=VERTEX_POINT('',#102406);
#29546=VERTEX_POINT('',#102408);
#29547=VERTEX_POINT('',#102412);
#29548=VERTEX_POINT('',#102414);
#29549=VERTEX_POINT('',#102418);
#29550=VERTEX_POINT('',#102422);
#29551=VERTEX_POINT('',#102426);
#29552=VERTEX_POINT('',#102427);
#29553=VERTEX_POINT('',#102429);
#29554=VERTEX_POINT('',#102431);
#29555=VERTEX_POINT('',#102435);
#29556=VERTEX_POINT('',#102437);
#29557=VERTEX_POINT('',#102441);
#29558=VERTEX_POINT('',#102445);
#29559=VERTEX_POINT('',#102449);
#29560=VERTEX_POINT('',#102450);
#29561=VERTEX_POINT('',#102452);
#29562=VERTEX_POINT('',#102454);
#29563=VERTEX_POINT('',#102458);
#29564=VERTEX_POINT('',#102460);
#29565=VERTEX_POINT('',#102464);
#29566=VERTEX_POINT('',#102468);
#29567=VERTEX_POINT('',#102472);
#29568=VERTEX_POINT('',#102473);
#29569=VERTEX_POINT('',#102475);
#29570=VERTEX_POINT('',#102477);
#29571=VERTEX_POINT('',#102481);
#29572=VERTEX_POINT('',#102483);
#29573=VERTEX_POINT('',#102487);
#29574=VERTEX_POINT('',#102491);
#29575=VERTEX_POINT('',#102495);
#29576=VERTEX_POINT('',#102496);
#29577=VERTEX_POINT('',#102500);
#29578=VERTEX_POINT('',#102502);
#29579=VERTEX_POINT('',#102506);
#29580=VERTEX_POINT('',#102507);
#29581=VERTEX_POINT('',#102511);
#29582=VERTEX_POINT('',#102513);
#29583=VERTEX_POINT('',#102520);
#29584=VERTEX_POINT('',#102524);
#29585=VERTEX_POINT('',#102543);
#29586=VERTEX_POINT('',#102547);
#29587=VERTEX_POINT('',#102549);
#29588=VERTEX_POINT('',#102551);
#29589=VERTEX_POINT('',#102553);
#29590=VERTEX_POINT('',#102555);
#29591=VERTEX_POINT('',#102562);
#29592=VERTEX_POINT('',#102564);
#29593=VERTEX_POINT('',#102568);
#29594=VERTEX_POINT('',#102571);
#29595=VERTEX_POINT('',#102573);
#29596=VERTEX_POINT('',#102579);
#29597=VERTEX_POINT('',#102583);
#29598=VERTEX_POINT('',#102585);
#29599=VERTEX_POINT('',#102589);
#29600=VERTEX_POINT('',#102591);
#29601=VERTEX_POINT('',#102595);
#29602=VERTEX_POINT('',#102598);
#29603=VERTEX_POINT('',#102604);
#29604=VERTEX_POINT('',#102606);
#29605=VERTEX_POINT('',#102610);
#29606=VERTEX_POINT('',#102611);
#29607=VERTEX_POINT('',#102616);
#29608=VERTEX_POINT('',#102620);
#37634=EDGE_CURVE('',#29447,#29448,#16198,.T.);
#37635=EDGE_CURVE('',#29449,#29447,#16199,.T.);
#37636=EDGE_CURVE('',#29449,#29450,#16200,.T.);
#37637=EDGE_CURVE('',#29450,#29448,#16201,.T.);
#37638=EDGE_CURVE('',#29448,#29451,#16202,.T.);
#37639=EDGE_CURVE('',#29452,#29450,#16203,.T.);
#37640=EDGE_CURVE('',#29451,#29452,#16204,.T.);
#37641=EDGE_CURVE('',#29453,#29449,#16205,.T.);
#37642=EDGE_CURVE('',#29453,#29452,#16206,.T.);
#37643=EDGE_CURVE('',#29451,#29454,#16207,.T.);
#37644=EDGE_CURVE('',#29454,#29453,#16208,.T.);
#37645=EDGE_CURVE('',#29455,#29456,#16209,.T.);
#37646=EDGE_CURVE('',#29457,#29455,#16210,.T.);
#37647=EDGE_CURVE('',#29457,#29458,#16211,.T.);
#37648=EDGE_CURVE('',#29458,#29456,#16212,.T.);
#37649=EDGE_CURVE('',#29456,#29459,#16213,.T.);
#37650=EDGE_CURVE('',#29460,#29458,#16214,.T.);
#37651=EDGE_CURVE('',#29459,#29460,#16215,.T.);
#37652=EDGE_CURVE('',#29461,#29457,#16216,.T.);
#37653=EDGE_CURVE('',#29461,#29460,#16217,.T.);
#37654=EDGE_CURVE('',#29459,#29462,#16218,.T.);
#37655=EDGE_CURVE('',#29462,#29461,#16219,.T.);
#37656=EDGE_CURVE('',#29463,#29464,#16220,.T.);
#37657=EDGE_CURVE('',#29465,#29463,#16221,.T.);
#37658=EDGE_CURVE('',#29465,#29466,#16222,.T.);
#37659=EDGE_CURVE('',#29466,#29464,#16223,.T.);
#37660=EDGE_CURVE('',#29464,#29467,#16224,.T.);
#37661=EDGE_CURVE('',#29468,#29466,#16225,.T.);
#37662=EDGE_CURVE('',#29467,#29468,#16226,.T.);
#37663=EDGE_CURVE('',#29469,#29465,#16227,.T.);
#37664=EDGE_CURVE('',#29469,#29468,#16228,.T.);
#37665=EDGE_CURVE('',#29467,#29470,#16229,.T.);
#37666=EDGE_CURVE('',#29470,#29469,#16230,.T.);
#37667=EDGE_CURVE('',#29471,#29472,#16231,.T.);
#37668=EDGE_CURVE('',#29473,#29471,#16232,.T.);
#37669=EDGE_CURVE('',#29473,#29474,#16233,.T.);
#37670=EDGE_CURVE('',#29474,#29472,#16234,.T.);
#37671=EDGE_CURVE('',#29472,#29475,#16235,.T.);
#37672=EDGE_CURVE('',#29476,#29474,#16236,.T.);
#37673=EDGE_CURVE('',#29475,#29476,#16237,.T.);
#37674=EDGE_CURVE('',#29477,#29473,#16238,.T.);
#37675=EDGE_CURVE('',#29477,#29476,#16239,.T.);
#37676=EDGE_CURVE('',#29475,#29478,#16240,.T.);
#37677=EDGE_CURVE('',#29478,#29477,#16241,.T.);
#37678=EDGE_CURVE('',#29479,#29480,#16242,.T.);
#37679=EDGE_CURVE('',#29481,#29479,#16243,.T.);
#37680=EDGE_CURVE('',#29481,#29482,#16244,.T.);
#37681=EDGE_CURVE('',#29482,#29480,#16245,.T.);
#37682=EDGE_CURVE('',#29480,#29483,#16246,.T.);
#37683=EDGE_CURVE('',#29484,#29482,#16247,.T.);
#37684=EDGE_CURVE('',#29483,#29484,#16248,.T.);
#37685=EDGE_CURVE('',#29485,#29481,#16249,.T.);
#37686=EDGE_CURVE('',#29485,#29484,#16250,.T.);
#37687=EDGE_CURVE('',#29483,#29486,#16251,.T.);
#37688=EDGE_CURVE('',#29486,#29485,#16252,.T.);
#37689=EDGE_CURVE('',#29487,#29488,#16253,.T.);
#37690=EDGE_CURVE('',#29489,#29487,#16254,.T.);
#37691=EDGE_CURVE('',#29489,#29490,#16255,.T.);
#37692=EDGE_CURVE('',#29490,#29488,#16256,.T.);
#37693=EDGE_CURVE('',#29488,#29491,#16257,.T.);
#37694=EDGE_CURVE('',#29492,#29490,#16258,.T.);
#37695=EDGE_CURVE('',#29491,#29492,#16259,.T.);
#37696=EDGE_CURVE('',#29493,#29489,#16260,.T.);
#37697=EDGE_CURVE('',#29493,#29492,#16261,.T.);
#37698=EDGE_CURVE('',#29491,#29494,#16262,.T.);
#37699=EDGE_CURVE('',#29494,#29493,#16263,.T.);
#37700=EDGE_CURVE('',#29495,#29496,#16264,.T.);
#37701=EDGE_CURVE('',#29497,#29495,#16265,.T.);
#37702=EDGE_CURVE('',#29497,#29498,#16266,.T.);
#37703=EDGE_CURVE('',#29498,#29496,#16267,.T.);
#37704=EDGE_CURVE('',#29496,#29499,#16268,.T.);
#37705=EDGE_CURVE('',#29500,#29498,#16269,.T.);
#37706=EDGE_CURVE('',#29499,#29500,#16270,.T.);
#37707=EDGE_CURVE('',#29501,#29497,#16271,.T.);
#37708=EDGE_CURVE('',#29501,#29500,#16272,.T.);
#37709=EDGE_CURVE('',#29499,#29502,#16273,.T.);
#37710=EDGE_CURVE('',#29502,#29501,#16274,.T.);
#37711=EDGE_CURVE('',#29503,#29504,#16275,.T.);
#37712=EDGE_CURVE('',#29505,#29503,#16276,.T.);
#37713=EDGE_CURVE('',#29505,#29506,#16277,.T.);
#37714=EDGE_CURVE('',#29506,#29504,#16278,.T.);
#37715=EDGE_CURVE('',#29504,#29507,#16279,.T.);
#37716=EDGE_CURVE('',#29508,#29506,#16280,.T.);
#37717=EDGE_CURVE('',#29507,#29508,#16281,.T.);
#37718=EDGE_CURVE('',#29509,#29505,#16282,.T.);
#37719=EDGE_CURVE('',#29509,#29508,#16283,.T.);
#37720=EDGE_CURVE('',#29507,#29510,#16284,.T.);
#37721=EDGE_CURVE('',#29510,#29509,#16285,.T.);
#37722=EDGE_CURVE('',#29511,#29512,#371,.T.);
#37723=EDGE_CURVE('',#29511,#29513,#16286,.T.);
#37724=EDGE_CURVE('',#29514,#29513,#16287,.T.);
#37725=EDGE_CURVE('',#29512,#29514,#16288,.T.);
#37726=EDGE_CURVE('',#29515,#29516,#372,.T.);
#37727=EDGE_CURVE('',#29517,#29515,#16289,.T.);
#37728=EDGE_CURVE('',#29518,#29517,#16290,.T.);
#37729=EDGE_CURVE('',#29518,#29516,#16291,.T.);
#37730=EDGE_CURVE('',#29516,#29511,#1266,.T.);
#37731=EDGE_CURVE('',#29513,#29518,#16292,.T.);
#37732=EDGE_CURVE('',#29519,#29520,#16293,.T.);
#37733=EDGE_CURVE('',#29521,#29519,#16294,.T.);
#37734=EDGE_CURVE('',#29521,#29522,#16295,.T.);
#37735=EDGE_CURVE('',#29522,#29520,#16296,.T.);
#37736=EDGE_CURVE('',#29520,#29523,#16297,.T.);
#37737=EDGE_CURVE('',#29524,#29522,#16298,.T.);
#37738=EDGE_CURVE('',#29523,#29524,#16299,.T.);
#37739=EDGE_CURVE('',#29525,#29521,#16300,.T.);
#37740=EDGE_CURVE('',#29525,#29524,#16301,.T.);
#37741=EDGE_CURVE('',#29523,#29526,#16302,.T.);
#37742=EDGE_CURVE('',#29526,#29525,#16303,.T.);
#37743=EDGE_CURVE('',#29527,#29528,#16304,.T.);
#37744=EDGE_CURVE('',#29529,#29527,#16305,.T.);
#37745=EDGE_CURVE('',#29529,#29530,#16306,.T.);
#37746=EDGE_CURVE('',#29530,#29528,#16307,.T.);
#37747=EDGE_CURVE('',#29528,#29531,#16308,.T.);
#37748=EDGE_CURVE('',#29532,#29530,#16309,.T.);
#37749=EDGE_CURVE('',#29531,#29532,#16310,.T.);
#37750=EDGE_CURVE('',#29533,#29529,#16311,.T.);
#37751=EDGE_CURVE('',#29533,#29532,#16312,.T.);
#37752=EDGE_CURVE('',#29531,#29534,#16313,.T.);
#37753=EDGE_CURVE('',#29534,#29533,#16314,.T.);
#37754=EDGE_CURVE('',#29535,#29536,#16315,.T.);
#37755=EDGE_CURVE('',#29537,#29535,#16316,.T.);
#37756=EDGE_CURVE('',#29537,#29538,#16317,.T.);
#37757=EDGE_CURVE('',#29538,#29536,#16318,.T.);
#37758=EDGE_CURVE('',#29536,#29539,#16319,.T.);
#37759=EDGE_CURVE('',#29540,#29538,#16320,.T.);
#37760=EDGE_CURVE('',#29539,#29540,#16321,.T.);
#37761=EDGE_CURVE('',#29541,#29537,#16322,.T.);
#37762=EDGE_CURVE('',#29541,#29540,#16323,.T.);
#37763=EDGE_CURVE('',#29539,#29542,#16324,.T.);
#37764=EDGE_CURVE('',#29542,#29541,#16325,.T.);
#37765=EDGE_CURVE('',#29543,#29544,#16326,.T.);
#37766=EDGE_CURVE('',#29545,#29543,#16327,.T.);
#37767=EDGE_CURVE('',#29545,#29546,#16328,.T.);
#37768=EDGE_CURVE('',#29546,#29544,#16329,.T.);
#37769=EDGE_CURVE('',#29544,#29547,#16330,.T.);
#37770=EDGE_CURVE('',#29548,#29546,#16331,.T.);
#37771=EDGE_CURVE('',#29547,#29548,#16332,.T.);
#37772=EDGE_CURVE('',#29549,#29545,#16333,.T.);
#37773=EDGE_CURVE('',#29549,#29548,#16334,.T.);
#37774=EDGE_CURVE('',#29547,#29550,#16335,.T.);
#37775=EDGE_CURVE('',#29550,#29549,#16336,.T.);
#37776=EDGE_CURVE('',#29551,#29552,#16337,.T.);
#37777=EDGE_CURVE('',#29553,#29551,#16338,.T.);
#37778=EDGE_CURVE('',#29553,#29554,#16339,.T.);
#37779=EDGE_CURVE('',#29554,#29552,#16340,.T.);
#37780=EDGE_CURVE('',#29552,#29555,#16341,.T.);
#37781=EDGE_CURVE('',#29556,#29554,#16342,.T.);
#37782=EDGE_CURVE('',#29555,#29556,#16343,.T.);
#37783=EDGE_CURVE('',#29557,#29553,#16344,.T.);
#37784=EDGE_CURVE('',#29557,#29556,#16345,.T.);
#37785=EDGE_CURVE('',#29555,#29558,#16346,.T.);
#37786=EDGE_CURVE('',#29558,#29557,#16347,.T.);
#37787=EDGE_CURVE('',#29559,#29560,#16348,.T.);
#37788=EDGE_CURVE('',#29561,#29559,#16349,.T.);
#37789=EDGE_CURVE('',#29561,#29562,#16350,.T.);
#37790=EDGE_CURVE('',#29562,#29560,#16351,.T.);
#37791=EDGE_CURVE('',#29560,#29563,#16352,.T.);
#37792=EDGE_CURVE('',#29564,#29562,#16353,.T.);
#37793=EDGE_CURVE('',#29563,#29564,#16354,.T.);
#37794=EDGE_CURVE('',#29565,#29561,#16355,.T.);
#37795=EDGE_CURVE('',#29565,#29564,#16356,.T.);
#37796=EDGE_CURVE('',#29563,#29566,#16357,.T.);
#37797=EDGE_CURVE('',#29566,#29565,#16358,.T.);
#37798=EDGE_CURVE('',#29567,#29568,#16359,.T.);
#37799=EDGE_CURVE('',#29569,#29567,#16360,.T.);
#37800=EDGE_CURVE('',#29569,#29570,#16361,.T.);
#37801=EDGE_CURVE('',#29570,#29568,#16362,.T.);
#37802=EDGE_CURVE('',#29568,#29571,#16363,.T.);
#37803=EDGE_CURVE('',#29572,#29570,#16364,.T.);
#37804=EDGE_CURVE('',#29571,#29572,#16365,.T.);
#37805=EDGE_CURVE('',#29573,#29569,#16366,.T.);
#37806=EDGE_CURVE('',#29573,#29572,#16367,.T.);
#37807=EDGE_CURVE('',#29571,#29574,#16368,.T.);
#37808=EDGE_CURVE('',#29574,#29573,#16369,.T.);
#37809=EDGE_CURVE('',#29575,#29576,#373,.T.);
#37810=EDGE_CURVE('',#29575,#29577,#16370,.T.);
#37811=EDGE_CURVE('',#29578,#29577,#16371,.T.);
#37812=EDGE_CURVE('',#29576,#29578,#16372,.T.);
#37813=EDGE_CURVE('',#29579,#29580,#374,.T.);
#37814=EDGE_CURVE('',#29581,#29579,#16373,.T.);
#37815=EDGE_CURVE('',#29582,#29581,#16374,.T.);
#37816=EDGE_CURVE('',#29582,#29580,#16375,.T.);
#37817=EDGE_CURVE('',#29580,#29575,#1267,.T.);
#37818=EDGE_CURVE('',#29577,#29582,#16376,.T.);
#37819=EDGE_CURVE('',#29578,#29583,#16377,.T.);
#37820=EDGE_CURVE('',#29583,#29576,#1268,.T.);
#37821=EDGE_CURVE('',#29515,#29584,#1269,.T.);
#37822=EDGE_CURVE('',#29584,#29517,#16378,.T.);
#37823=EDGE_CURVE('',#29567,#29454,#16379,.T.);
#37824=EDGE_CURVE('',#29455,#29574,#16380,.T.);
#37825=EDGE_CURVE('',#29559,#29462,#16381,.T.);
#37826=EDGE_CURVE('',#29463,#29566,#16382,.T.);
#37827=EDGE_CURVE('',#29551,#29470,#16383,.T.);
#37828=EDGE_CURVE('',#29471,#29558,#16384,.T.);
#37829=EDGE_CURVE('',#29479,#29478,#16385,.T.);
#37830=EDGE_CURVE('',#29543,#29486,#16386,.T.);
#37831=EDGE_CURVE('',#29487,#29550,#16387,.T.);
#37832=EDGE_CURVE('',#29535,#29494,#16388,.T.);
#37833=EDGE_CURVE('',#29495,#29542,#16389,.T.);
#37834=EDGE_CURVE('',#29527,#29502,#16390,.T.);
#37835=EDGE_CURVE('',#29503,#29534,#16391,.T.);
#37836=EDGE_CURVE('',#29519,#29510,#16392,.T.);
#37837=EDGE_CURVE('',#29514,#29526,#16393,.T.);
#37838=EDGE_CURVE('',#29584,#29585,#375,.T.);
#37839=EDGE_CURVE('',#29586,#29585,#16394,.T.);
#37840=EDGE_CURVE('',#29587,#29586,#16395,.T.);
#37841=EDGE_CURVE('',#29587,#29588,#16396,.T.);
#37842=EDGE_CURVE('',#29588,#29589,#16397,.T.);
#37843=EDGE_CURVE('',#29590,#29589,#16398,.T.);
#37844=EDGE_CURVE('',#29590,#29583,#376,.T.);
#37845=EDGE_CURVE('',#29447,#29581,#16399,.T.);
#37846=EDGE_CURVE('',#29591,#29591,#1270,.T.);
#37847=EDGE_CURVE('',#29591,#29592,#16400,.T.);
#37848=EDGE_CURVE('',#29592,#29592,#1271,.T.);
#37849=EDGE_CURVE('',#29592,#29593,#16401,.T.);
#37850=EDGE_CURVE('',#29579,#29593,#1272,.T.);
#37851=EDGE_CURVE('',#29594,#29590,#1273,.T.);
#37852=EDGE_CURVE('',#29595,#29594,#377,.T.);
#37853=EDGE_CURVE('',#29593,#29595,#1274,.T.);
#37854=EDGE_CURVE('',#29595,#29596,#16402,.T.);
#37855=EDGE_CURVE('',#29596,#29512,#1275,.T.);
#37856=EDGE_CURVE('',#29589,#29597,#16403,.T.);
#37857=EDGE_CURVE('',#29597,#29598,#1276,.T.);
#37858=EDGE_CURVE('',#29598,#29594,#16404,.T.);
#37859=EDGE_CURVE('',#29599,#29599,#1277,.T.);
#37860=EDGE_CURVE('',#29599,#29600,#16405,.T.);
#37861=EDGE_CURVE('',#29600,#29600,#1278,.T.);
#37862=EDGE_CURVE('',#29600,#29601,#16406,.T.);
#37863=EDGE_CURVE('',#29585,#29601,#1279,.T.);
#37864=EDGE_CURVE('',#29602,#29596,#378,.T.);
#37865=EDGE_CURVE('',#29601,#29602,#1280,.T.);
#37866=EDGE_CURVE('',#29602,#29603,#16407,.T.);
#37867=EDGE_CURVE('',#29603,#29604,#1281,.T.);
#37868=EDGE_CURVE('',#29604,#29586,#16408,.T.);
#37869=EDGE_CURVE('',#29605,#29606,#1282,.T.);
#37870=EDGE_CURVE('',#29606,#29604,#16409,.T.);
#37871=EDGE_CURVE('',#29605,#29603,#16410,.T.);
#37872=EDGE_CURVE('',#29607,#29598,#16411,.T.);
#37873=EDGE_CURVE('',#29607,#29605,#16412,.T.);
#37874=EDGE_CURVE('',#29608,#29607,#1283,.T.);
#37875=EDGE_CURVE('',#29608,#29597,#16413,.T.);
#37876=EDGE_CURVE('',#29588,#29608,#16414,.T.);
#37877=EDGE_CURVE('',#29606,#29587,#16415,.T.);
#53603=ORIENTED_EDGE('',*,*,#37634,.F.);
#53604=ORIENTED_EDGE('',*,*,#37635,.F.);
#53605=ORIENTED_EDGE('',*,*,#37636,.T.);
#53606=ORIENTED_EDGE('',*,*,#37637,.T.);
#53607=ORIENTED_EDGE('',*,*,#37638,.F.);
#53608=ORIENTED_EDGE('',*,*,#37637,.F.);
#53609=ORIENTED_EDGE('',*,*,#37639,.F.);
#53610=ORIENTED_EDGE('',*,*,#37640,.F.);
#53611=ORIENTED_EDGE('',*,*,#37641,.F.);
#53612=ORIENTED_EDGE('',*,*,#37642,.T.);
#53613=ORIENTED_EDGE('',*,*,#37639,.T.);
#53614=ORIENTED_EDGE('',*,*,#37636,.F.);
#53615=ORIENTED_EDGE('',*,*,#37643,.F.);
#53616=ORIENTED_EDGE('',*,*,#37640,.T.);
#53617=ORIENTED_EDGE('',*,*,#37642,.F.);
#53618=ORIENTED_EDGE('',*,*,#37644,.F.);
#53619=ORIENTED_EDGE('',*,*,#37645,.F.);
#53620=ORIENTED_EDGE('',*,*,#37646,.F.);
#53621=ORIENTED_EDGE('',*,*,#37647,.T.);
#53622=ORIENTED_EDGE('',*,*,#37648,.T.);
#53623=ORIENTED_EDGE('',*,*,#37649,.F.);
#53624=ORIENTED_EDGE('',*,*,#37648,.F.);
#53625=ORIENTED_EDGE('',*,*,#37650,.F.);
#53626=ORIENTED_EDGE('',*,*,#37651,.F.);
#53627=ORIENTED_EDGE('',*,*,#37652,.F.);
#53628=ORIENTED_EDGE('',*,*,#37653,.T.);
#53629=ORIENTED_EDGE('',*,*,#37650,.T.);
#53630=ORIENTED_EDGE('',*,*,#37647,.F.);
#53631=ORIENTED_EDGE('',*,*,#37654,.F.);
#53632=ORIENTED_EDGE('',*,*,#37651,.T.);
#53633=ORIENTED_EDGE('',*,*,#37653,.F.);
#53634=ORIENTED_EDGE('',*,*,#37655,.F.);
#53635=ORIENTED_EDGE('',*,*,#37656,.F.);
#53636=ORIENTED_EDGE('',*,*,#37657,.F.);
#53637=ORIENTED_EDGE('',*,*,#37658,.T.);
#53638=ORIENTED_EDGE('',*,*,#37659,.T.);
#53639=ORIENTED_EDGE('',*,*,#37660,.F.);
#53640=ORIENTED_EDGE('',*,*,#37659,.F.);
#53641=ORIENTED_EDGE('',*,*,#37661,.F.);
#53642=ORIENTED_EDGE('',*,*,#37662,.F.);
#53643=ORIENTED_EDGE('',*,*,#37663,.F.);
#53644=ORIENTED_EDGE('',*,*,#37664,.T.);
#53645=ORIENTED_EDGE('',*,*,#37661,.T.);
#53646=ORIENTED_EDGE('',*,*,#37658,.F.);
#53647=ORIENTED_EDGE('',*,*,#37665,.F.);
#53648=ORIENTED_EDGE('',*,*,#37662,.T.);
#53649=ORIENTED_EDGE('',*,*,#37664,.F.);
#53650=ORIENTED_EDGE('',*,*,#37666,.F.);
#53651=ORIENTED_EDGE('',*,*,#37667,.F.);
#53652=ORIENTED_EDGE('',*,*,#37668,.F.);
#53653=ORIENTED_EDGE('',*,*,#37669,.T.);
#53654=ORIENTED_EDGE('',*,*,#37670,.T.);
#53655=ORIENTED_EDGE('',*,*,#37671,.F.);
#53656=ORIENTED_EDGE('',*,*,#37670,.F.);
#53657=ORIENTED_EDGE('',*,*,#37672,.F.);
#53658=ORIENTED_EDGE('',*,*,#37673,.F.);
#53659=ORIENTED_EDGE('',*,*,#37674,.F.);
#53660=ORIENTED_EDGE('',*,*,#37675,.T.);
#53661=ORIENTED_EDGE('',*,*,#37672,.T.);
#53662=ORIENTED_EDGE('',*,*,#37669,.F.);
#53663=ORIENTED_EDGE('',*,*,#37676,.F.);
#53664=ORIENTED_EDGE('',*,*,#37673,.T.);
#53665=ORIENTED_EDGE('',*,*,#37675,.F.);
#53666=ORIENTED_EDGE('',*,*,#37677,.F.);
#53667=ORIENTED_EDGE('',*,*,#37678,.F.);
#53668=ORIENTED_EDGE('',*,*,#37679,.F.);
#53669=ORIENTED_EDGE('',*,*,#37680,.T.);
#53670=ORIENTED_EDGE('',*,*,#37681,.T.);
#53671=ORIENTED_EDGE('',*,*,#37682,.F.);
#53672=ORIENTED_EDGE('',*,*,#37681,.F.);
#53673=ORIENTED_EDGE('',*,*,#37683,.F.);
#53674=ORIENTED_EDGE('',*,*,#37684,.F.);
#53675=ORIENTED_EDGE('',*,*,#37685,.F.);
#53676=ORIENTED_EDGE('',*,*,#37686,.T.);
#53677=ORIENTED_EDGE('',*,*,#37683,.T.);
#53678=ORIENTED_EDGE('',*,*,#37680,.F.);
#53679=ORIENTED_EDGE('',*,*,#37687,.F.);
#53680=ORIENTED_EDGE('',*,*,#37684,.T.);
#53681=ORIENTED_EDGE('',*,*,#37686,.F.);
#53682=ORIENTED_EDGE('',*,*,#37688,.F.);
#53683=ORIENTED_EDGE('',*,*,#37689,.F.);
#53684=ORIENTED_EDGE('',*,*,#37690,.F.);
#53685=ORIENTED_EDGE('',*,*,#37691,.T.);
#53686=ORIENTED_EDGE('',*,*,#37692,.T.);
#53687=ORIENTED_EDGE('',*,*,#37693,.F.);
#53688=ORIENTED_EDGE('',*,*,#37692,.F.);
#53689=ORIENTED_EDGE('',*,*,#37694,.F.);
#53690=ORIENTED_EDGE('',*,*,#37695,.F.);
#53691=ORIENTED_EDGE('',*,*,#37696,.F.);
#53692=ORIENTED_EDGE('',*,*,#37697,.T.);
#53693=ORIENTED_EDGE('',*,*,#37694,.T.);
#53694=ORIENTED_EDGE('',*,*,#37691,.F.);
#53695=ORIENTED_EDGE('',*,*,#37698,.F.);
#53696=ORIENTED_EDGE('',*,*,#37695,.T.);
#53697=ORIENTED_EDGE('',*,*,#37697,.F.);
#53698=ORIENTED_EDGE('',*,*,#37699,.F.);
#53699=ORIENTED_EDGE('',*,*,#37700,.F.);
#53700=ORIENTED_EDGE('',*,*,#37701,.F.);
#53701=ORIENTED_EDGE('',*,*,#37702,.T.);
#53702=ORIENTED_EDGE('',*,*,#37703,.T.);
#53703=ORIENTED_EDGE('',*,*,#37704,.F.);
#53704=ORIENTED_EDGE('',*,*,#37703,.F.);
#53705=ORIENTED_EDGE('',*,*,#37705,.F.);
#53706=ORIENTED_EDGE('',*,*,#37706,.F.);
#53707=ORIENTED_EDGE('',*,*,#37707,.F.);
#53708=ORIENTED_EDGE('',*,*,#37708,.T.);
#53709=ORIENTED_EDGE('',*,*,#37705,.T.);
#53710=ORIENTED_EDGE('',*,*,#37702,.F.);
#53711=ORIENTED_EDGE('',*,*,#37709,.F.);
#53712=ORIENTED_EDGE('',*,*,#37706,.T.);
#53713=ORIENTED_EDGE('',*,*,#37708,.F.);
#53714=ORIENTED_EDGE('',*,*,#37710,.F.);
#53715=ORIENTED_EDGE('',*,*,#37711,.F.);
#53716=ORIENTED_EDGE('',*,*,#37712,.F.);
#53717=ORIENTED_EDGE('',*,*,#37713,.T.);
#53718=ORIENTED_EDGE('',*,*,#37714,.T.);
#53719=ORIENTED_EDGE('',*,*,#37715,.F.);
#53720=ORIENTED_EDGE('',*,*,#37714,.F.);
#53721=ORIENTED_EDGE('',*,*,#37716,.F.);
#53722=ORIENTED_EDGE('',*,*,#37717,.F.);
#53723=ORIENTED_EDGE('',*,*,#37718,.F.);
#53724=ORIENTED_EDGE('',*,*,#37719,.T.);
#53725=ORIENTED_EDGE('',*,*,#37716,.T.);
#53726=ORIENTED_EDGE('',*,*,#37713,.F.);
#53727=ORIENTED_EDGE('',*,*,#37720,.F.);
#53728=ORIENTED_EDGE('',*,*,#37717,.T.);
#53729=ORIENTED_EDGE('',*,*,#37719,.F.);
#53730=ORIENTED_EDGE('',*,*,#37721,.F.);
#53731=ORIENTED_EDGE('',*,*,#37722,.F.);
#53732=ORIENTED_EDGE('',*,*,#37723,.T.);
#53733=ORIENTED_EDGE('',*,*,#37724,.F.);
#53734=ORIENTED_EDGE('',*,*,#37725,.F.);
#53735=ORIENTED_EDGE('',*,*,#37726,.F.);
#53736=ORIENTED_EDGE('',*,*,#37727,.F.);
#53737=ORIENTED_EDGE('',*,*,#37728,.F.);
#53738=ORIENTED_EDGE('',*,*,#37729,.T.);
#53739=ORIENTED_EDGE('',*,*,#37730,.F.);
#53740=ORIENTED_EDGE('',*,*,#37729,.F.);
#53741=ORIENTED_EDGE('',*,*,#37731,.F.);
#53742=ORIENTED_EDGE('',*,*,#37723,.F.);
#53743=ORIENTED_EDGE('',*,*,#37732,.F.);
#53744=ORIENTED_EDGE('',*,*,#37733,.F.);
#53745=ORIENTED_EDGE('',*,*,#37734,.T.);
#53746=ORIENTED_EDGE('',*,*,#37735,.T.);
#53747=ORIENTED_EDGE('',*,*,#37736,.F.);
#53748=ORIENTED_EDGE('',*,*,#37735,.F.);
#53749=ORIENTED_EDGE('',*,*,#37737,.F.);
#53750=ORIENTED_EDGE('',*,*,#37738,.F.);
#53751=ORIENTED_EDGE('',*,*,#37739,.F.);
#53752=ORIENTED_EDGE('',*,*,#37740,.T.);
#53753=ORIENTED_EDGE('',*,*,#37737,.T.);
#53754=ORIENTED_EDGE('',*,*,#37734,.F.);
#53755=ORIENTED_EDGE('',*,*,#37741,.F.);
#53756=ORIENTED_EDGE('',*,*,#37738,.T.);
#53757=ORIENTED_EDGE('',*,*,#37740,.F.);
#53758=ORIENTED_EDGE('',*,*,#37742,.F.);
#53759=ORIENTED_EDGE('',*,*,#37743,.F.);
#53760=ORIENTED_EDGE('',*,*,#37744,.F.);
#53761=ORIENTED_EDGE('',*,*,#37745,.T.);
#53762=ORIENTED_EDGE('',*,*,#37746,.T.);
#53763=ORIENTED_EDGE('',*,*,#37747,.F.);
#53764=ORIENTED_EDGE('',*,*,#37746,.F.);
#53765=ORIENTED_EDGE('',*,*,#37748,.F.);
#53766=ORIENTED_EDGE('',*,*,#37749,.F.);
#53767=ORIENTED_EDGE('',*,*,#37750,.F.);
#53768=ORIENTED_EDGE('',*,*,#37751,.T.);
#53769=ORIENTED_EDGE('',*,*,#37748,.T.);
#53770=ORIENTED_EDGE('',*,*,#37745,.F.);
#53771=ORIENTED_EDGE('',*,*,#37752,.F.);
#53772=ORIENTED_EDGE('',*,*,#37749,.T.);
#53773=ORIENTED_EDGE('',*,*,#37751,.F.);
#53774=ORIENTED_EDGE('',*,*,#37753,.F.);
#53775=ORIENTED_EDGE('',*,*,#37754,.F.);
#53776=ORIENTED_EDGE('',*,*,#37755,.F.);
#53777=ORIENTED_EDGE('',*,*,#37756,.T.);
#53778=ORIENTED_EDGE('',*,*,#37757,.T.);
#53779=ORIENTED_EDGE('',*,*,#37758,.F.);
#53780=ORIENTED_EDGE('',*,*,#37757,.F.);
#53781=ORIENTED_EDGE('',*,*,#37759,.F.);
#53782=ORIENTED_EDGE('',*,*,#37760,.F.);
#53783=ORIENTED_EDGE('',*,*,#37761,.F.);
#53784=ORIENTED_EDGE('',*,*,#37762,.T.);
#53785=ORIENTED_EDGE('',*,*,#37759,.T.);
#53786=ORIENTED_EDGE('',*,*,#37756,.F.);
#53787=ORIENTED_EDGE('',*,*,#37763,.F.);
#53788=ORIENTED_EDGE('',*,*,#37760,.T.);
#53789=ORIENTED_EDGE('',*,*,#37762,.F.);
#53790=ORIENTED_EDGE('',*,*,#37764,.F.);
#53791=ORIENTED_EDGE('',*,*,#37765,.F.);
#53792=ORIENTED_EDGE('',*,*,#37766,.F.);
#53793=ORIENTED_EDGE('',*,*,#37767,.T.);
#53794=ORIENTED_EDGE('',*,*,#37768,.T.);
#53795=ORIENTED_EDGE('',*,*,#37769,.F.);
#53796=ORIENTED_EDGE('',*,*,#37768,.F.);
#53797=ORIENTED_EDGE('',*,*,#37770,.F.);
#53798=ORIENTED_EDGE('',*,*,#37771,.F.);
#53799=ORIENTED_EDGE('',*,*,#37772,.F.);
#53800=ORIENTED_EDGE('',*,*,#37773,.T.);
#53801=ORIENTED_EDGE('',*,*,#37770,.T.);
#53802=ORIENTED_EDGE('',*,*,#37767,.F.);
#53803=ORIENTED_EDGE('',*,*,#37774,.F.);
#53804=ORIENTED_EDGE('',*,*,#37771,.T.);
#53805=ORIENTED_EDGE('',*,*,#37773,.F.);
#53806=ORIENTED_EDGE('',*,*,#37775,.F.);
#53807=ORIENTED_EDGE('',*,*,#37776,.F.);
#53808=ORIENTED_EDGE('',*,*,#37777,.F.);
#53809=ORIENTED_EDGE('',*,*,#37778,.T.);
#53810=ORIENTED_EDGE('',*,*,#37779,.T.);
#53811=ORIENTED_EDGE('',*,*,#37780,.F.);
#53812=ORIENTED_EDGE('',*,*,#37779,.F.);
#53813=ORIENTED_EDGE('',*,*,#37781,.F.);
#53814=ORIENTED_EDGE('',*,*,#37782,.F.);
#53815=ORIENTED_EDGE('',*,*,#37783,.F.);
#53816=ORIENTED_EDGE('',*,*,#37784,.T.);
#53817=ORIENTED_EDGE('',*,*,#37781,.T.);
#53818=ORIENTED_EDGE('',*,*,#37778,.F.);
#53819=ORIENTED_EDGE('',*,*,#37785,.F.);
#53820=ORIENTED_EDGE('',*,*,#37782,.T.);
#53821=ORIENTED_EDGE('',*,*,#37784,.F.);
#53822=ORIENTED_EDGE('',*,*,#37786,.F.);
#53823=ORIENTED_EDGE('',*,*,#37787,.F.);
#53824=ORIENTED_EDGE('',*,*,#37788,.F.);
#53825=ORIENTED_EDGE('',*,*,#37789,.T.);
#53826=ORIENTED_EDGE('',*,*,#37790,.T.);
#53827=ORIENTED_EDGE('',*,*,#37791,.F.);
#53828=ORIENTED_EDGE('',*,*,#37790,.F.);
#53829=ORIENTED_EDGE('',*,*,#37792,.F.);
#53830=ORIENTED_EDGE('',*,*,#37793,.F.);
#53831=ORIENTED_EDGE('',*,*,#37794,.F.);
#53832=ORIENTED_EDGE('',*,*,#37795,.T.);
#53833=ORIENTED_EDGE('',*,*,#37792,.T.);
#53834=ORIENTED_EDGE('',*,*,#37789,.F.);
#53835=ORIENTED_EDGE('',*,*,#37796,.F.);
#53836=ORIENTED_EDGE('',*,*,#37793,.T.);
#53837=ORIENTED_EDGE('',*,*,#37795,.F.);
#53838=ORIENTED_EDGE('',*,*,#37797,.F.);
#53839=ORIENTED_EDGE('',*,*,#37798,.F.);
#53840=ORIENTED_EDGE('',*,*,#37799,.F.);
#53841=ORIENTED_EDGE('',*,*,#37800,.T.);
#53842=ORIENTED_EDGE('',*,*,#37801,.T.);
#53843=ORIENTED_EDGE('',*,*,#37802,.F.);
#53844=ORIENTED_EDGE('',*,*,#37801,.F.);
#53845=ORIENTED_EDGE('',*,*,#37803,.F.);
#53846=ORIENTED_EDGE('',*,*,#37804,.F.);
#53847=ORIENTED_EDGE('',*,*,#37805,.F.);
#53848=ORIENTED_EDGE('',*,*,#37806,.T.);
#53849=ORIENTED_EDGE('',*,*,#37803,.T.);
#53850=ORIENTED_EDGE('',*,*,#37800,.F.);
#53851=ORIENTED_EDGE('',*,*,#37807,.F.);
#53852=ORIENTED_EDGE('',*,*,#37804,.T.);
#53853=ORIENTED_EDGE('',*,*,#37806,.F.);
#53854=ORIENTED_EDGE('',*,*,#37808,.F.);
#53855=ORIENTED_EDGE('',*,*,#37809,.F.);
#53856=ORIENTED_EDGE('',*,*,#37810,.T.);
#53857=ORIENTED_EDGE('',*,*,#37811,.F.);
#53858=ORIENTED_EDGE('',*,*,#37812,.F.);
#53859=ORIENTED_EDGE('',*,*,#37813,.F.);
#53860=ORIENTED_EDGE('',*,*,#37814,.F.);
#53861=ORIENTED_EDGE('',*,*,#37815,.F.);
#53862=ORIENTED_EDGE('',*,*,#37816,.T.);
#53863=ORIENTED_EDGE('',*,*,#37817,.F.);
#53864=ORIENTED_EDGE('',*,*,#37816,.F.);
#53865=ORIENTED_EDGE('',*,*,#37818,.F.);
#53866=ORIENTED_EDGE('',*,*,#37810,.F.);
#53867=ORIENTED_EDGE('',*,*,#37812,.T.);
#53868=ORIENTED_EDGE('',*,*,#37819,.T.);
#53869=ORIENTED_EDGE('',*,*,#37820,.T.);
#53870=ORIENTED_EDGE('',*,*,#37727,.T.);
#53871=ORIENTED_EDGE('',*,*,#37821,.T.);
#53872=ORIENTED_EDGE('',*,*,#37822,.T.);
#53873=ORIENTED_EDGE('',*,*,#37634,.T.);
#53874=ORIENTED_EDGE('',*,*,#37638,.T.);
#53875=ORIENTED_EDGE('',*,*,#37643,.T.);
#53876=ORIENTED_EDGE('',*,*,#37823,.F.);
#53877=ORIENTED_EDGE('',*,*,#37798,.T.);
#53878=ORIENTED_EDGE('',*,*,#37802,.T.);
#53879=ORIENTED_EDGE('',*,*,#37807,.T.);
#53880=ORIENTED_EDGE('',*,*,#37824,.F.);
#53881=ORIENTED_EDGE('',*,*,#37645,.T.);
#53882=ORIENTED_EDGE('',*,*,#37649,.T.);
#53883=ORIENTED_EDGE('',*,*,#37654,.T.);
#53884=ORIENTED_EDGE('',*,*,#37825,.F.);
#53885=ORIENTED_EDGE('',*,*,#37787,.T.);
#53886=ORIENTED_EDGE('',*,*,#37791,.T.);
#53887=ORIENTED_EDGE('',*,*,#37796,.T.);
#53888=ORIENTED_EDGE('',*,*,#37826,.F.);
#53889=ORIENTED_EDGE('',*,*,#37656,.T.);
#53890=ORIENTED_EDGE('',*,*,#37660,.T.);
#53891=ORIENTED_EDGE('',*,*,#37665,.T.);
#53892=ORIENTED_EDGE('',*,*,#37827,.F.);
#53893=ORIENTED_EDGE('',*,*,#37776,.T.);
#53894=ORIENTED_EDGE('',*,*,#37780,.T.);
#53895=ORIENTED_EDGE('',*,*,#37785,.T.);
#53896=ORIENTED_EDGE('',*,*,#37828,.F.);
#53897=ORIENTED_EDGE('',*,*,#37667,.T.);
#53898=ORIENTED_EDGE('',*,*,#37671,.T.);
#53899=ORIENTED_EDGE('',*,*,#37676,.T.);
#53900=ORIENTED_EDGE('',*,*,#37829,.F.);
#53901=ORIENTED_EDGE('',*,*,#37678,.T.);
#53902=ORIENTED_EDGE('',*,*,#37682,.T.);
#53903=ORIENTED_EDGE('',*,*,#37687,.T.);
#53904=ORIENTED_EDGE('',*,*,#37830,.F.);
#53905=ORIENTED_EDGE('',*,*,#37765,.T.);
#53906=ORIENTED_EDGE('',*,*,#37769,.T.);
#53907=ORIENTED_EDGE('',*,*,#37774,.T.);
#53908=ORIENTED_EDGE('',*,*,#37831,.F.);
#53909=ORIENTED_EDGE('',*,*,#37689,.T.);
#53910=ORIENTED_EDGE('',*,*,#37693,.T.);
#53911=ORIENTED_EDGE('',*,*,#37698,.T.);
#53912=ORIENTED_EDGE('',*,*,#37832,.F.);
#53913=ORIENTED_EDGE('',*,*,#37754,.T.);
#53914=ORIENTED_EDGE('',*,*,#37758,.T.);
#53915=ORIENTED_EDGE('',*,*,#37763,.T.);
#53916=ORIENTED_EDGE('',*,*,#37833,.F.);
#53917=ORIENTED_EDGE('',*,*,#37700,.T.);
#53918=ORIENTED_EDGE('',*,*,#37704,.T.);
#53919=ORIENTED_EDGE('',*,*,#37709,.T.);
#53920=ORIENTED_EDGE('',*,*,#37834,.F.);
#53921=ORIENTED_EDGE('',*,*,#37743,.T.);
#53922=ORIENTED_EDGE('',*,*,#37747,.T.);
#53923=ORIENTED_EDGE('',*,*,#37752,.T.);
#53924=ORIENTED_EDGE('',*,*,#37835,.F.);
#53925=ORIENTED_EDGE('',*,*,#37711,.T.);
#53926=ORIENTED_EDGE('',*,*,#37715,.T.);
#53927=ORIENTED_EDGE('',*,*,#37720,.T.);
#53928=ORIENTED_EDGE('',*,*,#37836,.F.);
#53929=ORIENTED_EDGE('',*,*,#37732,.T.);
#53930=ORIENTED_EDGE('',*,*,#37736,.T.);
#53931=ORIENTED_EDGE('',*,*,#37741,.T.);
#53932=ORIENTED_EDGE('',*,*,#37837,.F.);
#53933=ORIENTED_EDGE('',*,*,#37724,.T.);
#53934=ORIENTED_EDGE('',*,*,#37731,.T.);
#53935=ORIENTED_EDGE('',*,*,#37728,.T.);
#53936=ORIENTED_EDGE('',*,*,#37822,.F.);
#53937=ORIENTED_EDGE('',*,*,#37838,.T.);
#53938=ORIENTED_EDGE('',*,*,#37839,.F.);
#53939=ORIENTED_EDGE('',*,*,#37840,.F.);
#53940=ORIENTED_EDGE('',*,*,#37841,.T.);
#53941=ORIENTED_EDGE('',*,*,#37842,.T.);
#53942=ORIENTED_EDGE('',*,*,#37843,.F.);
#53943=ORIENTED_EDGE('',*,*,#37844,.T.);
#53944=ORIENTED_EDGE('',*,*,#37819,.F.);
#53945=ORIENTED_EDGE('',*,*,#37811,.T.);
#53946=ORIENTED_EDGE('',*,*,#37818,.T.);
#53947=ORIENTED_EDGE('',*,*,#37815,.T.);
#53948=ORIENTED_EDGE('',*,*,#37845,.F.);
#53949=ORIENTED_EDGE('',*,*,#37846,.F.);
#53950=ORIENTED_EDGE('',*,*,#37847,.T.);
#53951=ORIENTED_EDGE('',*,*,#37848,.T.);
#53952=ORIENTED_EDGE('',*,*,#37847,.F.);
#53953=ORIENTED_EDGE('',*,*,#37848,.F.);
#53954=ORIENTED_EDGE('',*,*,#37849,.T.);
#53955=ORIENTED_EDGE('',*,*,#37850,.F.);
#53956=ORIENTED_EDGE('',*,*,#37813,.T.);
#53957=ORIENTED_EDGE('',*,*,#37817,.T.);
#53958=ORIENTED_EDGE('',*,*,#37809,.T.);
#53959=ORIENTED_EDGE('',*,*,#37820,.F.);
#53960=ORIENTED_EDGE('',*,*,#37844,.F.);
#53961=ORIENTED_EDGE('',*,*,#37851,.F.);
#53962=ORIENTED_EDGE('',*,*,#37852,.F.);
#53963=ORIENTED_EDGE('',*,*,#37853,.F.);
#53964=ORIENTED_EDGE('',*,*,#37849,.F.);
#53965=ORIENTED_EDGE('',*,*,#37635,.T.);
#53966=ORIENTED_EDGE('',*,*,#37845,.T.);
#53967=ORIENTED_EDGE('',*,*,#37814,.T.);
#53968=ORIENTED_EDGE('',*,*,#37850,.T.);
#53969=ORIENTED_EDGE('',*,*,#37853,.T.);
#53970=ORIENTED_EDGE('',*,*,#37854,.T.);
#53971=ORIENTED_EDGE('',*,*,#37855,.T.);
#53972=ORIENTED_EDGE('',*,*,#37725,.T.);
#53973=ORIENTED_EDGE('',*,*,#37837,.T.);
#53974=ORIENTED_EDGE('',*,*,#37742,.T.);
#53975=ORIENTED_EDGE('',*,*,#37739,.T.);
#53976=ORIENTED_EDGE('',*,*,#37733,.T.);
#53977=ORIENTED_EDGE('',*,*,#37836,.T.);
#53978=ORIENTED_EDGE('',*,*,#37721,.T.);
#53979=ORIENTED_EDGE('',*,*,#37718,.T.);
#53980=ORIENTED_EDGE('',*,*,#37712,.T.);
#53981=ORIENTED_EDGE('',*,*,#37835,.T.);
#53982=ORIENTED_EDGE('',*,*,#37753,.T.);
#53983=ORIENTED_EDGE('',*,*,#37750,.T.);
#53984=ORIENTED_EDGE('',*,*,#37744,.T.);
#53985=ORIENTED_EDGE('',*,*,#37834,.T.);
#53986=ORIENTED_EDGE('',*,*,#37710,.T.);
#53987=ORIENTED_EDGE('',*,*,#37707,.T.);
#53988=ORIENTED_EDGE('',*,*,#37701,.T.);
#53989=ORIENTED_EDGE('',*,*,#37833,.T.);
#53990=ORIENTED_EDGE('',*,*,#37764,.T.);
#53991=ORIENTED_EDGE('',*,*,#37761,.T.);
#53992=ORIENTED_EDGE('',*,*,#37755,.T.);
#53993=ORIENTED_EDGE('',*,*,#37832,.T.);
#53994=ORIENTED_EDGE('',*,*,#37699,.T.);
#53995=ORIENTED_EDGE('',*,*,#37696,.T.);
#53996=ORIENTED_EDGE('',*,*,#37690,.T.);
#53997=ORIENTED_EDGE('',*,*,#37831,.T.);
#53998=ORIENTED_EDGE('',*,*,#37775,.T.);
#53999=ORIENTED_EDGE('',*,*,#37772,.T.);
#54000=ORIENTED_EDGE('',*,*,#37766,.T.);
#54001=ORIENTED_EDGE('',*,*,#37830,.T.);
#54002=ORIENTED_EDGE('',*,*,#37688,.T.);
#54003=ORIENTED_EDGE('',*,*,#37685,.T.);
#54004=ORIENTED_EDGE('',*,*,#37679,.T.);
#54005=ORIENTED_EDGE('',*,*,#37829,.T.);
#54006=ORIENTED_EDGE('',*,*,#37677,.T.);
#54007=ORIENTED_EDGE('',*,*,#37674,.T.);
#54008=ORIENTED_EDGE('',*,*,#37668,.T.);
#54009=ORIENTED_EDGE('',*,*,#37828,.T.);
#54010=ORIENTED_EDGE('',*,*,#37786,.T.);
#54011=ORIENTED_EDGE('',*,*,#37783,.T.);
#54012=ORIENTED_EDGE('',*,*,#37777,.T.);
#54013=ORIENTED_EDGE('',*,*,#37827,.T.);
#54014=ORIENTED_EDGE('',*,*,#37666,.T.);
#54015=ORIENTED_EDGE('',*,*,#37663,.T.);
#54016=ORIENTED_EDGE('',*,*,#37657,.T.);
#54017=ORIENTED_EDGE('',*,*,#37826,.T.);
#54018=ORIENTED_EDGE('',*,*,#37797,.T.);
#54019=ORIENTED_EDGE('',*,*,#37794,.T.);
#54020=ORIENTED_EDGE('',*,*,#37788,.T.);
#54021=ORIENTED_EDGE('',*,*,#37825,.T.);
#54022=ORIENTED_EDGE('',*,*,#37655,.T.);
#54023=ORIENTED_EDGE('',*,*,#37652,.T.);
#54024=ORIENTED_EDGE('',*,*,#37646,.T.);
#54025=ORIENTED_EDGE('',*,*,#37824,.T.);
#54026=ORIENTED_EDGE('',*,*,#37808,.T.);
#54027=ORIENTED_EDGE('',*,*,#37805,.T.);
#54028=ORIENTED_EDGE('',*,*,#37799,.T.);
#54029=ORIENTED_EDGE('',*,*,#37823,.T.);
#54030=ORIENTED_EDGE('',*,*,#37644,.T.);
#54031=ORIENTED_EDGE('',*,*,#37641,.T.);
#54032=ORIENTED_EDGE('',*,*,#37851,.T.);
#54033=ORIENTED_EDGE('',*,*,#37843,.T.);
#54034=ORIENTED_EDGE('',*,*,#37856,.T.);
#54035=ORIENTED_EDGE('',*,*,#37857,.T.);
#54036=ORIENTED_EDGE('',*,*,#37858,.T.);
#54037=ORIENTED_EDGE('',*,*,#37859,.F.);
#54038=ORIENTED_EDGE('',*,*,#37860,.T.);
#54039=ORIENTED_EDGE('',*,*,#37861,.T.);
#54040=ORIENTED_EDGE('',*,*,#37860,.F.);
#54041=ORIENTED_EDGE('',*,*,#37861,.F.);
#54042=ORIENTED_EDGE('',*,*,#37862,.T.);
#54043=ORIENTED_EDGE('',*,*,#37863,.F.);
#54044=ORIENTED_EDGE('',*,*,#37838,.F.);
#54045=ORIENTED_EDGE('',*,*,#37821,.F.);
#54046=ORIENTED_EDGE('',*,*,#37726,.T.);
#54047=ORIENTED_EDGE('',*,*,#37730,.T.);
#54048=ORIENTED_EDGE('',*,*,#37722,.T.);
#54049=ORIENTED_EDGE('',*,*,#37855,.F.);
#54050=ORIENTED_EDGE('',*,*,#37864,.F.);
#54051=ORIENTED_EDGE('',*,*,#37865,.F.);
#54052=ORIENTED_EDGE('',*,*,#37862,.F.);
#54053=ORIENTED_EDGE('',*,*,#37863,.T.);
#54054=ORIENTED_EDGE('',*,*,#37865,.T.);
#54055=ORIENTED_EDGE('',*,*,#37866,.T.);
#54056=ORIENTED_EDGE('',*,*,#37867,.T.);
#54057=ORIENTED_EDGE('',*,*,#37868,.T.);
#54058=ORIENTED_EDGE('',*,*,#37839,.T.);
#54059=ORIENTED_EDGE('',*,*,#37869,.T.);
#54060=ORIENTED_EDGE('',*,*,#37870,.T.);
#54061=ORIENTED_EDGE('',*,*,#37867,.F.);
#54062=ORIENTED_EDGE('',*,*,#37871,.F.);
#54063=ORIENTED_EDGE('',*,*,#37852,.T.);
#54064=ORIENTED_EDGE('',*,*,#37858,.F.);
#54065=ORIENTED_EDGE('',*,*,#37872,.F.);
#54066=ORIENTED_EDGE('',*,*,#37873,.T.);
#54067=ORIENTED_EDGE('',*,*,#37871,.T.);
#54068=ORIENTED_EDGE('',*,*,#37866,.F.);
#54069=ORIENTED_EDGE('',*,*,#37864,.T.);
#54070=ORIENTED_EDGE('',*,*,#37854,.F.);
#54071=ORIENTED_EDGE('',*,*,#37874,.T.);
#54072=ORIENTED_EDGE('',*,*,#37872,.T.);
#54073=ORIENTED_EDGE('',*,*,#37857,.F.);
#54074=ORIENTED_EDGE('',*,*,#37875,.F.);
#54075=ORIENTED_EDGE('',*,*,#37876,.T.);
#54076=ORIENTED_EDGE('',*,*,#37875,.T.);
#54077=ORIENTED_EDGE('',*,*,#37856,.F.);
#54078=ORIENTED_EDGE('',*,*,#37842,.F.);
#54079=ORIENTED_EDGE('',*,*,#37877,.T.);
#54080=ORIENTED_EDGE('',*,*,#37840,.T.);
#54081=ORIENTED_EDGE('',*,*,#37868,.F.);
#54082=ORIENTED_EDGE('',*,*,#37870,.F.);
#54083=ORIENTED_EDGE('',*,*,#37877,.F.);
#54084=ORIENTED_EDGE('',*,*,#37869,.F.);
#54085=ORIENTED_EDGE('',*,*,#37873,.F.);
#54086=ORIENTED_EDGE('',*,*,#37874,.F.);
#54087=ORIENTED_EDGE('',*,*,#37876,.F.);
#54088=ORIENTED_EDGE('',*,*,#37841,.F.);
#54089=ORIENTED_EDGE('',*,*,#37846,.T.);
#54090=ORIENTED_EDGE('',*,*,#37859,.T.);
#59868=ADVANCED_FACE('',(#6768),#3708,.F.);
#59869=ADVANCED_FACE('',(#6769),#3709,.F.);
#59870=ADVANCED_FACE('',(#6770),#3710,.F.);
#59871=ADVANCED_FACE('',(#6771),#3711,.F.);
#59872=ADVANCED_FACE('',(#6772),#3712,.F.);
#59873=ADVANCED_FACE('',(#6773),#3713,.F.);
#59874=ADVANCED_FACE('',(#6774),#3714,.F.);
#59875=ADVANCED_FACE('',(#6775),#3715,.F.);
#59876=ADVANCED_FACE('',(#6776),#3716,.F.);
#59877=ADVANCED_FACE('',(#6777),#3717,.F.);
#59878=ADVANCED_FACE('',(#6778),#3718,.F.);
#59879=ADVANCED_FACE('',(#6779),#3719,.F.);
#59880=ADVANCED_FACE('',(#6780),#3720,.F.);
#59881=ADVANCED_FACE('',(#6781),#3721,.F.);
#59882=ADVANCED_FACE('',(#6782),#3722,.F.);
#59883=ADVANCED_FACE('',(#6783),#3723,.F.);
#59884=ADVANCED_FACE('',(#6784),#3724,.F.);
#59885=ADVANCED_FACE('',(#6785),#3725,.F.);
#59886=ADVANCED_FACE('',(#6786),#3726,.F.);
#59887=ADVANCED_FACE('',(#6787),#3727,.F.);
#59888=ADVANCED_FACE('',(#6788),#3728,.F.);
#59889=ADVANCED_FACE('',(#6789),#3729,.F.);
#59890=ADVANCED_FACE('',(#6790),#3730,.F.);
#59891=ADVANCED_FACE('',(#6791),#3731,.F.);
#59892=ADVANCED_FACE('',(#6792),#3732,.F.);
#59893=ADVANCED_FACE('',(#6793),#3733,.F.);
#59894=ADVANCED_FACE('',(#6794),#3734,.F.);
#59895=ADVANCED_FACE('',(#6795),#3735,.F.);
#59896=ADVANCED_FACE('',(#6796),#3736,.F.);
#59897=ADVANCED_FACE('',(#6797),#3737,.F.);
#59898=ADVANCED_FACE('',(#6798),#3738,.F.);
#59899=ADVANCED_FACE('',(#6799),#3739,.F.);
#59900=ADVANCED_FACE('',(#6800),#3740,.F.);
#59901=ADVANCED_FACE('',(#6801),#3741,.F.);
#59902=ADVANCED_FACE('',(#6802),#3742,.F.);
#59903=ADVANCED_FACE('',(#6803),#3743,.F.);
#59904=ADVANCED_FACE('',(#6804),#3744,.F.);
#59905=ADVANCED_FACE('',(#6805),#3745,.F.);
#59906=ADVANCED_FACE('',(#6806),#3746,.F.);
#59907=ADVANCED_FACE('',(#6807),#3747,.F.);
#59908=ADVANCED_FACE('',(#6808),#3748,.F.);
#59909=ADVANCED_FACE('',(#6809),#3749,.F.);
#59910=ADVANCED_FACE('',(#6810),#3750,.F.);
#59911=ADVANCED_FACE('',(#6811),#3751,.F.);
#59912=ADVANCED_FACE('',(#6812),#3752,.F.);
#59913=ADVANCED_FACE('',(#6813),#3753,.F.);
#59914=ADVANCED_FACE('',(#6814),#3754,.F.);
#59915=ADVANCED_FACE('',(#6815),#3755,.F.);
#59916=ADVANCED_FACE('',(#6816),#3756,.F.);
#59917=ADVANCED_FACE('',(#6817),#3757,.F.);
#59918=ADVANCED_FACE('',(#6818),#3758,.F.);
#59919=ADVANCED_FACE('',(#6819),#3759,.F.);
#59920=ADVANCED_FACE('',(#6820),#3760,.F.);
#59921=ADVANCED_FACE('',(#6821),#3761,.F.);
#59922=ADVANCED_FACE('',(#6822),#3762,.F.);
#59923=ADVANCED_FACE('',(#6823),#3763,.F.);
#59924=ADVANCED_FACE('',(#6824),#3764,.F.);
#59925=ADVANCED_FACE('',(#6825),#3765,.F.);
#59926=ADVANCED_FACE('',(#6826),#3766,.F.);
#59927=ADVANCED_FACE('',(#6827),#3767,.F.);
#59928=ADVANCED_FACE('',(#6828),#3768,.F.);
#59929=ADVANCED_FACE('',(#6829),#3769,.F.);
#59930=ADVANCED_FACE('',(#6830),#3770,.F.);
#59931=ADVANCED_FACE('',(#6831),#3771,.F.);
#59932=ADVANCED_FACE('',(#6832),#3772,.F.);
#59933=ADVANCED_FACE('',(#6833),#3773,.F.);
#59934=ADVANCED_FACE('',(#6834),#3774,.T.);
#59935=ADVANCED_FACE('',(#6835),#3775,.T.);
#59936=ADVANCED_FACE('',(#6836),#3776,.T.);
#59937=ADVANCED_FACE('',(#6837),#714,.F.);
#59938=ADVANCED_FACE('',(#6838),#928,.F.);
#59939=ADVANCED_FACE('',(#6839),#3777,.T.);
#59940=ADVANCED_FACE('',(#6840),#3778,.T.);
#59941=ADVANCED_FACE('',(#6841),#715,.F.);
#59942=ADVANCED_FACE('',(#6842),#929,.F.);
#59943=ADVANCED_FACE('',(#6843),#3779,.T.);
#59944=ADVANCED_FACE('',(#6844),#716,.T.);
#59945=ADVANCED_FACE('',(#6845),#3780,.T.);
#59946=ADVANCED_FACE('',(#6846),#717,.T.);
#59947=ADVANCED_FACE('',(#6847),#3781,.T.);
#59948=ADVANCED_FACE('',(#6848),#3782,.T.);
#59949=ADVANCED_FACE('',(#6849,#1849,#1850),#3783,.F.);
#60401=CLOSED_SHELL('',(#59868,#59869,#59870,#59871,#59872,#59873,#59874,
#59875,#59876,#59877,#59878,#59879,#59880,#59881,#59882,#59883,#59884,#59885,
#59886,#59887,#59888,#59889,#59890,#59891,#59892,#59893,#59894,#59895,#59896,
#59897,#59898,#59899,#59900,#59901,#59902,#59903,#59904,#59905,#59906,#59907,
#59908,#59909,#59910,#59911,#59912,#59913,#59914,#59915,#59916,#59917,#59918,
#59919,#59920,#59921,#59922,#59923,#59924,#59925,#59926,#59927,#59928,#59929,
#59930,#59931,#59932,#59933,#59934,#59935,#59936,#59937,#59938,#59939,#59940,
#59941,#59942,#59943,#59944,#59945,#59946,#59947,#59948,#59949));
#62957=AXIS2_PLACEMENT_3D('',#102123,#73794,#73795);
#62958=AXIS2_PLACEMENT_3D('',#102124,#73796,#73797);
#62959=AXIS2_PLACEMENT_3D('',#102133,#73802,#73803);
#62960=AXIS2_PLACEMENT_3D('',#102139,#73807,#73808);
#62961=AXIS2_PLACEMENT_3D('',#102143,#73811,#73812);
#62962=AXIS2_PLACEMENT_3D('',#102147,#73815,#73816);
#62963=AXIS2_PLACEMENT_3D('',#102156,#73821,#73822);
#62964=AXIS2_PLACEMENT_3D('',#102162,#73826,#73827);
#62965=AXIS2_PLACEMENT_3D('',#102166,#73830,#73831);
#62966=AXIS2_PLACEMENT_3D('',#102170,#73834,#73835);
#62967=AXIS2_PLACEMENT_3D('',#102179,#73840,#73841);
#62968=AXIS2_PLACEMENT_3D('',#102185,#73845,#73846);
#62969=AXIS2_PLACEMENT_3D('',#102189,#73849,#73850);
#62970=AXIS2_PLACEMENT_3D('',#102193,#73853,#73854);
#62971=AXIS2_PLACEMENT_3D('',#102202,#73859,#73860);
#62972=AXIS2_PLACEMENT_3D('',#102208,#73864,#73865);
#62973=AXIS2_PLACEMENT_3D('',#102212,#73868,#73869);
#62974=AXIS2_PLACEMENT_3D('',#102216,#73872,#73873);
#62975=AXIS2_PLACEMENT_3D('',#102225,#73878,#73879);
#62976=AXIS2_PLACEMENT_3D('',#102231,#73883,#73884);
#62977=AXIS2_PLACEMENT_3D('',#102235,#73887,#73888);
#62978=AXIS2_PLACEMENT_3D('',#102239,#73891,#73892);
#62979=AXIS2_PLACEMENT_3D('',#102248,#73897,#73898);
#62980=AXIS2_PLACEMENT_3D('',#102254,#73902,#73903);
#62981=AXIS2_PLACEMENT_3D('',#102258,#73906,#73907);
#62982=AXIS2_PLACEMENT_3D('',#102262,#73910,#73911);
#62983=AXIS2_PLACEMENT_3D('',#102271,#73916,#73917);
#62984=AXIS2_PLACEMENT_3D('',#102277,#73921,#73922);
#62985=AXIS2_PLACEMENT_3D('',#102281,#73925,#73926);
#62986=AXIS2_PLACEMENT_3D('',#102285,#73929,#73930);
#62987=AXIS2_PLACEMENT_3D('',#102294,#73935,#73936);
#62988=AXIS2_PLACEMENT_3D('',#102300,#73940,#73941);
#62989=AXIS2_PLACEMENT_3D('',#102304,#73944,#73945);
#62990=AXIS2_PLACEMENT_3D('',#102308,#73948,#73949);
#62991=AXIS2_PLACEMENT_3D('',#102319,#73953,#73954);
#62992=AXIS2_PLACEMENT_3D('',#102330,#73958,#73959);
#62993=AXIS2_PLACEMENT_3D('',#102331,#73960,#73961);
#62994=AXIS2_PLACEMENT_3D('',#102333,#73963,#73964);
#62995=AXIS2_PLACEMENT_3D('',#102342,#73969,#73970);
#62996=AXIS2_PLACEMENT_3D('',#102348,#73974,#73975);
#62997=AXIS2_PLACEMENT_3D('',#102352,#73978,#73979);
#62998=AXIS2_PLACEMENT_3D('',#102356,#73982,#73983);
#62999=AXIS2_PLACEMENT_3D('',#102365,#73988,#73989);
#63000=AXIS2_PLACEMENT_3D('',#102371,#73993,#73994);
#63001=AXIS2_PLACEMENT_3D('',#102375,#73997,#73998);
#63002=AXIS2_PLACEMENT_3D('',#102379,#74001,#74002);
#63003=AXIS2_PLACEMENT_3D('',#102388,#74007,#74008);
#63004=AXIS2_PLACEMENT_3D('',#102394,#74012,#74013);
#63005=AXIS2_PLACEMENT_3D('',#102398,#74016,#74017);
#63006=AXIS2_PLACEMENT_3D('',#102402,#74020,#74021);
#63007=AXIS2_PLACEMENT_3D('',#102411,#74026,#74027);
#63008=AXIS2_PLACEMENT_3D('',#102417,#74031,#74032);
#63009=AXIS2_PLACEMENT_3D('',#102421,#74035,#74036);
#63010=AXIS2_PLACEMENT_3D('',#102425,#74039,#74040);
#63011=AXIS2_PLACEMENT_3D('',#102434,#74045,#74046);
#63012=AXIS2_PLACEMENT_3D('',#102440,#74050,#74051);
#63013=AXIS2_PLACEMENT_3D('',#102444,#74054,#74055);
#63014=AXIS2_PLACEMENT_3D('',#102448,#74058,#74059);
#63015=AXIS2_PLACEMENT_3D('',#102457,#74064,#74065);
#63016=AXIS2_PLACEMENT_3D('',#102463,#74069,#74070);
#63017=AXIS2_PLACEMENT_3D('',#102467,#74073,#74074);
#63018=AXIS2_PLACEMENT_3D('',#102471,#74077,#74078);
#63019=AXIS2_PLACEMENT_3D('',#102480,#74083,#74084);
#63020=AXIS2_PLACEMENT_3D('',#102486,#74088,#74089);
#63021=AXIS2_PLACEMENT_3D('',#102490,#74092,#74093);
#63022=AXIS2_PLACEMENT_3D('',#102494,#74096,#74097);
#63023=AXIS2_PLACEMENT_3D('',#102505,#74101,#74102);
#63024=AXIS2_PLACEMENT_3D('',#102516,#74106,#74107);
#63025=AXIS2_PLACEMENT_3D('',#102517,#74108,#74109);
#63026=AXIS2_PLACEMENT_3D('',#102519,#74111,#74112);
#63027=AXIS2_PLACEMENT_3D('',#102522,#74114,#74115);
#63028=AXIS2_PLACEMENT_3D('',#102523,#74116,#74117);
#63029=AXIS2_PLACEMENT_3D('',#102525,#74118,#74119);
#63030=AXIS2_PLACEMENT_3D('',#102527,#74121,#74122);
#63031=AXIS2_PLACEMENT_3D('',#102561,#74144,#74145);
#63032=AXIS2_PLACEMENT_3D('',#102563,#74146,#74147);
#63033=AXIS2_PLACEMENT_3D('',#102566,#74149,#74150);
#63034=AXIS2_PLACEMENT_3D('',#102567,#74151,#74152);
#63035=AXIS2_PLACEMENT_3D('',#102570,#74154,#74155);
#63036=AXIS2_PLACEMENT_3D('',#102572,#74156,#74157);
#63037=AXIS2_PLACEMENT_3D('',#102577,#74158,#74159);
#63038=AXIS2_PLACEMENT_3D('',#102578,#74160,#74161);
#63039=AXIS2_PLACEMENT_3D('',#102581,#74163,#74164);
#63040=AXIS2_PLACEMENT_3D('',#102582,#74165,#74166);
#63041=AXIS2_PLACEMENT_3D('',#102586,#74168,#74169);
#63042=AXIS2_PLACEMENT_3D('',#102588,#74171,#74172);
#63043=AXIS2_PLACEMENT_3D('',#102590,#74173,#74174);
#63044=AXIS2_PLACEMENT_3D('',#102593,#74176,#74177);
#63045=AXIS2_PLACEMENT_3D('',#102594,#74178,#74179);
#63046=AXIS2_PLACEMENT_3D('',#102597,#74181,#74182);
#63047=AXIS2_PLACEMENT_3D('',#102602,#74183,#74184);
#63048=AXIS2_PLACEMENT_3D('',#102603,#74185,#74186);
#63049=AXIS2_PLACEMENT_3D('',#102607,#74188,#74189);
#63050=AXIS2_PLACEMENT_3D('',#102609,#74191,#74192);
#63051=AXIS2_PLACEMENT_3D('',#102612,#74193,#74194);
#63052=AXIS2_PLACEMENT_3D('',#102615,#74197,#74198);
#63053=AXIS2_PLACEMENT_3D('',#102619,#74201,#74202);
#63054=AXIS2_PLACEMENT_3D('',#102621,#74203,#74204);
#63055=AXIS2_PLACEMENT_3D('',#102623,#74206,#74207);
#63056=AXIS2_PLACEMENT_3D('',#102625,#74209,#74210);
#63057=AXIS2_PLACEMENT_3D('',#102627,#74212,#74213);
#73794=DIRECTION('axis',(0.,0.,1.));
#73795=DIRECTION('refdir',(1.,0.,0.));
#73796=DIRECTION('center_axis',(1.,0.,0.));
#73797=DIRECTION('ref_axis',(0.,-1.,0.));
#73798=DIRECTION('',(0.,0.,-1.));
#73799=DIRECTION('',(0.,-1.,0.));
#73800=DIRECTION('',(0.,0.,-1.));
#73801=DIRECTION('',(0.,-1.,0.));
#73802=DIRECTION('center_axis',(0.,0.,-1.));
#73803=DIRECTION('ref_axis',(-1.,0.,0.));
#73804=DIRECTION('',(-1.,0.,0.));
#73805=DIRECTION('',(1.,0.,0.));
#73806=DIRECTION('',(0.,1.,0.));
#73807=DIRECTION('center_axis',(0.,1.,0.));
#73808=DIRECTION('ref_axis',(1.,0.,0.));
#73809=DIRECTION('',(1.,0.,0.));
#73810=DIRECTION('',(0.,0.,-1.));
#73811=DIRECTION('center_axis',(-1.,0.,0.));
#73812=DIRECTION('ref_axis',(0.,1.,0.));
#73813=DIRECTION('',(0.,0.,1.));
#73814=DIRECTION('',(0.,1.,0.));
#73815=DIRECTION('center_axis',(1.,0.,0.));
#73816=DIRECTION('ref_axis',(0.,-1.,0.));
#73817=DIRECTION('',(0.,0.,-1.));
#73818=DIRECTION('',(0.,-1.,0.));
#73819=DIRECTION('',(0.,0.,-1.));
#73820=DIRECTION('',(0.,-1.,0.));
#73821=DIRECTION('center_axis',(0.,0.,-1.));
#73822=DIRECTION('ref_axis',(-1.,0.,0.));
#73823=DIRECTION('',(-1.,0.,0.));
#73824=DIRECTION('',(1.,0.,0.));
#73825=DIRECTION('',(0.,1.,0.));
#73826=DIRECTION('center_axis',(0.,1.,0.));
#73827=DIRECTION('ref_axis',(1.,0.,0.));
#73828=DIRECTION('',(1.,0.,0.));
#73829=DIRECTION('',(0.,0.,-1.));
#73830=DIRECTION('center_axis',(-1.,0.,0.));
#73831=DIRECTION('ref_axis',(0.,1.,0.));
#73832=DIRECTION('',(0.,0.,1.));
#73833=DIRECTION('',(0.,1.,0.));
#73834=DIRECTION('center_axis',(1.,0.,0.));
#73835=DIRECTION('ref_axis',(0.,-1.,0.));
#73836=DIRECTION('',(0.,0.,-1.));
#73837=DIRECTION('',(0.,-1.,0.));
#73838=DIRECTION('',(0.,0.,-1.));
#73839=DIRECTION('',(0.,-1.,0.));
#73840=DIRECTION('center_axis',(0.,0.,-1.));
#73841=DIRECTION('ref_axis',(-1.,0.,0.));
#73842=DIRECTION('',(-1.,0.,0.));
#73843=DIRECTION('',(1.,0.,0.));
#73844=DIRECTION('',(0.,1.,0.));
#73845=DIRECTION('center_axis',(0.,1.,0.));
#73846=DIRECTION('ref_axis',(1.,0.,0.));
#73847=DIRECTION('',(1.,0.,0.));
#73848=DIRECTION('',(0.,0.,-1.));
#73849=DIRECTION('center_axis',(-1.,0.,0.));
#73850=DIRECTION('ref_axis',(0.,1.,0.));
#73851=DIRECTION('',(0.,0.,1.));
#73852=DIRECTION('',(0.,1.,0.));
#73853=DIRECTION('center_axis',(1.,0.,0.));
#73854=DIRECTION('ref_axis',(0.,-1.,0.));
#73855=DIRECTION('',(0.,0.,-1.));
#73856=DIRECTION('',(0.,-1.,0.));
#73857=DIRECTION('',(0.,0.,-1.));
#73858=DIRECTION('',(0.,-1.,0.));
#73859=DIRECTION('center_axis',(0.,0.,-1.));
#73860=DIRECTION('ref_axis',(-1.,0.,0.));
#73861=DIRECTION('',(-1.,0.,0.));
#73862=DIRECTION('',(1.,0.,0.));
#73863=DIRECTION('',(0.,1.,0.));
#73864=DIRECTION('center_axis',(0.,1.,0.));
#73865=DIRECTION('ref_axis',(1.,0.,0.));
#73866=DIRECTION('',(1.,0.,0.));
#73867=DIRECTION('',(0.,0.,-1.));
#73868=DIRECTION('center_axis',(-1.,0.,0.));
#73869=DIRECTION('ref_axis',(0.,1.,0.));
#73870=DIRECTION('',(0.,0.,1.));
#73871=DIRECTION('',(0.,1.,0.));
#73872=DIRECTION('center_axis',(1.,0.,0.));
#73873=DIRECTION('ref_axis',(0.,-1.,0.));
#73874=DIRECTION('',(0.,0.,-1.));
#73875=DIRECTION('',(0.,-1.,0.));
#73876=DIRECTION('',(0.,0.,-1.));
#73877=DIRECTION('',(0.,-1.,0.));
#73878=DIRECTION('center_axis',(0.,0.,-1.));
#73879=DIRECTION('ref_axis',(-1.,0.,0.));
#73880=DIRECTION('',(-1.,0.,0.));
#73881=DIRECTION('',(1.,0.,0.));
#73882=DIRECTION('',(0.,1.,0.));
#73883=DIRECTION('center_axis',(0.,1.,0.));
#73884=DIRECTION('ref_axis',(1.,0.,0.));
#73885=DIRECTION('',(1.,0.,0.));
#73886=DIRECTION('',(0.,0.,-1.));
#73887=DIRECTION('center_axis',(-1.,0.,0.));
#73888=DIRECTION('ref_axis',(0.,1.,0.));
#73889=DIRECTION('',(0.,0.,1.));
#73890=DIRECTION('',(0.,1.,0.));
#73891=DIRECTION('center_axis',(1.,0.,0.));
#73892=DIRECTION('ref_axis',(0.,-1.,0.));
#73893=DIRECTION('',(0.,0.,-1.));
#73894=DIRECTION('',(0.,-1.,0.));
#73895=DIRECTION('',(0.,0.,-1.));
#73896=DIRECTION('',(0.,-1.,0.));
#73897=DIRECTION('center_axis',(0.,0.,-1.));
#73898=DIRECTION('ref_axis',(-1.,0.,0.));
#73899=DIRECTION('',(-1.,0.,0.));
#73900=DIRECTION('',(1.,0.,0.));
#73901=DIRECTION('',(0.,1.,0.));
#73902=DIRECTION('center_axis',(0.,1.,0.));
#73903=DIRECTION('ref_axis',(1.,0.,0.));
#73904=DIRECTION('',(1.,0.,0.));
#73905=DIRECTION('',(0.,0.,-1.));
#73906=DIRECTION('center_axis',(-1.,0.,0.));
#73907=DIRECTION('ref_axis',(0.,1.,0.));
#73908=DIRECTION('',(0.,0.,1.));
#73909=DIRECTION('',(0.,1.,0.));
#73910=DIRECTION('center_axis',(1.,0.,0.));
#73911=DIRECTION('ref_axis',(0.,-1.,0.));
#73912=DIRECTION('',(0.,0.,-1.));
#73913=DIRECTION('',(0.,-1.,0.));
#73914=DIRECTION('',(0.,0.,-1.));
#73915=DIRECTION('',(0.,-1.,0.));
#73916=DIRECTION('center_axis',(0.,0.,-1.));
#73917=DIRECTION('ref_axis',(-1.,0.,0.));
#73918=DIRECTION('',(-1.,0.,0.));
#73919=DIRECTION('',(1.,0.,0.));
#73920=DIRECTION('',(0.,1.,0.));
#73921=DIRECTION('center_axis',(0.,1.,0.));
#73922=DIRECTION('ref_axis',(1.,0.,0.));
#73923=DIRECTION('',(1.,0.,0.));
#73924=DIRECTION('',(0.,0.,-1.));
#73925=DIRECTION('center_axis',(-1.,0.,0.));
#73926=DIRECTION('ref_axis',(0.,1.,0.));
#73927=DIRECTION('',(0.,0.,1.));
#73928=DIRECTION('',(0.,1.,0.));
#73929=DIRECTION('center_axis',(1.,0.,0.));
#73930=DIRECTION('ref_axis',(0.,-1.,0.));
#73931=DIRECTION('',(0.,0.,-1.));
#73932=DIRECTION('',(0.,-1.,0.));
#73933=DIRECTION('',(0.,0.,-1.));
#73934=DIRECTION('',(0.,-1.,0.));
#73935=DIRECTION('center_axis',(0.,0.,-1.));
#73936=DIRECTION('ref_axis',(-1.,0.,0.));
#73937=DIRECTION('',(-1.,0.,0.));
#73938=DIRECTION('',(1.,0.,0.));
#73939=DIRECTION('',(0.,1.,0.));
#73940=DIRECTION('center_axis',(0.,1.,0.));
#73941=DIRECTION('ref_axis',(1.,0.,0.));
#73942=DIRECTION('',(1.,0.,0.));
#73943=DIRECTION('',(0.,0.,-1.));
#73944=DIRECTION('center_axis',(-1.,0.,0.));
#73945=DIRECTION('ref_axis',(0.,1.,0.));
#73946=DIRECTION('',(0.,0.,1.));
#73947=DIRECTION('',(0.,1.,0.));
#73948=DIRECTION('center_axis',(1.,0.,0.));
#73949=DIRECTION('ref_axis',(0.,-1.,0.));
#73950=DIRECTION('',(0.,-1.,0.));
#73951=DIRECTION('',(0.,0.,-1.));
#73952=DIRECTION('',(0.,-1.,0.));
#73953=DIRECTION('center_axis',(-1.,0.,0.));
#73954=DIRECTION('ref_axis',(0.,1.,0.));
#73955=DIRECTION('',(0.,1.,0.));
#73956=DIRECTION('',(0.,0.,1.));
#73957=DIRECTION('',(0.,1.,0.));
#73958=DIRECTION('center_axis',(0.,0.,-1.));
#73959=DIRECTION('ref_axis',(-1.,0.,0.));
#73960=DIRECTION('center_axis',(0.,0.,1.));
#73961=DIRECTION('ref_axis',(1.,0.,0.));
#73962=DIRECTION('',(-1.,0.,0.));
#73963=DIRECTION('center_axis',(1.,0.,0.));
#73964=DIRECTION('ref_axis',(0.,-1.,0.));
#73965=DIRECTION('',(0.,0.,-1.));
#73966=DIRECTION('',(0.,-1.,0.));
#73967=DIRECTION('',(0.,0.,-1.));
#73968=DIRECTION('',(0.,-1.,0.));
#73969=DIRECTION('center_axis',(0.,0.,-1.));
#73970=DIRECTION('ref_axis',(-1.,0.,0.));
#73971=DIRECTION('',(-1.,0.,0.));
#73972=DIRECTION('',(1.,0.,0.));
#73973=DIRECTION('',(0.,1.,0.));
#73974=DIRECTION('center_axis',(0.,1.,0.));
#73975=DIRECTION('ref_axis',(1.,0.,0.));
#73976=DIRECTION('',(1.,0.,0.));
#73977=DIRECTION('',(0.,0.,-1.));
#73978=DIRECTION('center_axis',(-1.,0.,0.));
#73979=DIRECTION('ref_axis',(0.,1.,0.));
#73980=DIRECTION('',(0.,0.,1.));
#73981=DIRECTION('',(0.,1.,0.));
#73982=DIRECTION('center_axis',(1.,0.,0.));
#73983=DIRECTION('ref_axis',(0.,-1.,0.));
#73984=DIRECTION('',(0.,0.,-1.));
#73985=DIRECTION('',(0.,-1.,0.));
#73986=DIRECTION('',(0.,0.,-1.));
#73987=DIRECTION('',(0.,-1.,0.));
#73988=DIRECTION('center_axis',(0.,0.,-1.));
#73989=DIRECTION('ref_axis',(-1.,0.,0.));
#73990=DIRECTION('',(-1.,0.,0.));
#73991=DIRECTION('',(1.,0.,0.));
#73992=DIRECTION('',(0.,1.,0.));
#73993=DIRECTION('center_axis',(0.,1.,0.));
#73994=DIRECTION('ref_axis',(1.,0.,0.));
#73995=DIRECTION('',(1.,0.,0.));
#73996=DIRECTION('',(0.,0.,-1.));
#73997=DIRECTION('center_axis',(-1.,0.,0.));
#73998=DIRECTION('ref_axis',(0.,1.,0.));
#73999=DIRECTION('',(0.,0.,1.));
#74000=DIRECTION('',(0.,1.,0.));
#74001=DIRECTION('center_axis',(1.,0.,0.));
#74002=DIRECTION('ref_axis',(0.,-1.,0.));
#74003=DIRECTION('',(0.,0.,-1.));
#74004=DIRECTION('',(0.,-1.,0.));
#74005=DIRECTION('',(0.,0.,-1.));
#74006=DIRECTION('',(0.,-1.,0.));
#74007=DIRECTION('center_axis',(0.,0.,-1.));
#74008=DIRECTION('ref_axis',(-1.,0.,0.));
#74009=DIRECTION('',(-1.,0.,0.));
#74010=DIRECTION('',(1.,0.,0.));
#74011=DIRECTION('',(0.,1.,0.));
#74012=DIRECTION('center_axis',(0.,1.,0.));
#74013=DIRECTION('ref_axis',(1.,0.,0.));
#74014=DIRECTION('',(1.,0.,0.));
#74015=DIRECTION('',(0.,0.,-1.));
#74016=DIRECTION('center_axis',(-1.,0.,0.));
#74017=DIRECTION('ref_axis',(0.,1.,0.));
#74018=DIRECTION('',(0.,0.,1.));
#74019=DIRECTION('',(0.,1.,0.));
#74020=DIRECTION('center_axis',(1.,0.,0.));
#74021=DIRECTION('ref_axis',(0.,-1.,0.));
#74022=DIRECTION('',(0.,0.,-1.));
#74023=DIRECTION('',(0.,-1.,0.));
#74024=DIRECTION('',(0.,0.,-1.));
#74025=DIRECTION('',(0.,-1.,0.));
#74026=DIRECTION('center_axis',(0.,0.,-1.));
#74027=DIRECTION('ref_axis',(-1.,0.,0.));
#74028=DIRECTION('',(-1.,0.,0.));
#74029=DIRECTION('',(1.,0.,0.));
#74030=DIRECTION('',(0.,1.,0.));
#74031=DIRECTION('center_axis',(0.,1.,0.));
#74032=DIRECTION('ref_axis',(1.,0.,0.));
#74033=DIRECTION('',(1.,0.,0.));
#74034=DIRECTION('',(0.,0.,-1.));
#74035=DIRECTION('center_axis',(-1.,0.,0.));
#74036=DIRECTION('ref_axis',(0.,1.,0.));
#74037=DIRECTION('',(0.,0.,1.));
#74038=DIRECTION('',(0.,1.,0.));
#74039=DIRECTION('center_axis',(1.,0.,0.));
#74040=DIRECTION('ref_axis',(0.,-1.,0.));
#74041=DIRECTION('',(0.,0.,-1.));
#74042=DIRECTION('',(0.,-1.,0.));
#74043=DIRECTION('',(0.,0.,-1.));
#74044=DIRECTION('',(0.,-1.,0.));
#74045=DIRECTION('center_axis',(0.,0.,-1.));
#74046=DIRECTION('ref_axis',(-1.,0.,0.));
#74047=DIRECTION('',(-1.,0.,0.));
#74048=DIRECTION('',(1.,0.,0.));
#74049=DIRECTION('',(0.,1.,0.));
#74050=DIRECTION('center_axis',(0.,1.,0.));
#74051=DIRECTION('ref_axis',(1.,0.,0.));
#74052=DIRECTION('',(1.,0.,0.));
#74053=DIRECTION('',(0.,0.,-1.));
#74054=DIRECTION('center_axis',(-1.,0.,0.));
#74055=DIRECTION('ref_axis',(0.,1.,0.));
#74056=DIRECTION('',(0.,0.,1.));
#74057=DIRECTION('',(0.,1.,0.));
#74058=DIRECTION('center_axis',(1.,0.,0.));
#74059=DIRECTION('ref_axis',(0.,-1.,0.));
#74060=DIRECTION('',(0.,0.,-1.));
#74061=DIRECTION('',(0.,-1.,0.));
#74062=DIRECTION('',(0.,0.,-1.));
#74063=DIRECTION('',(0.,-1.,0.));
#74064=DIRECTION('center_axis',(0.,0.,-1.));
#74065=DIRECTION('ref_axis',(-1.,0.,0.));
#74066=DIRECTION('',(-1.,0.,0.));
#74067=DIRECTION('',(1.,0.,0.));
#74068=DIRECTION('',(0.,1.,0.));
#74069=DIRECTION('center_axis',(0.,1.,0.));
#74070=DIRECTION('ref_axis',(1.,0.,0.));
#74071=DIRECTION('',(1.,0.,0.));
#74072=DIRECTION('',(0.,0.,-1.));
#74073=DIRECTION('center_axis',(-1.,0.,0.));
#74074=DIRECTION('ref_axis',(0.,1.,0.));
#74075=DIRECTION('',(0.,0.,1.));
#74076=DIRECTION('',(0.,1.,0.));
#74077=DIRECTION('center_axis',(1.,0.,0.));
#74078=DIRECTION('ref_axis',(0.,-1.,0.));
#74079=DIRECTION('',(0.,0.,-1.));
#74080=DIRECTION('',(0.,-1.,0.));
#74081=DIRECTION('',(0.,0.,-1.));
#74082=DIRECTION('',(0.,-1.,0.));
#74083=DIRECTION('center_axis',(0.,0.,-1.));
#74084=DIRECTION('ref_axis',(-1.,0.,0.));
#74085=DIRECTION('',(-1.,0.,0.));
#74086=DIRECTION('',(1.,0.,0.));
#74087=DIRECTION('',(0.,1.,0.));
#74088=DIRECTION('center_axis',(0.,1.,0.));
#74089=DIRECTION('ref_axis',(1.,0.,0.));
#74090=DIRECTION('',(1.,0.,0.));
#74091=DIRECTION('',(0.,0.,-1.));
#74092=DIRECTION('center_axis',(-1.,0.,0.));
#74093=DIRECTION('ref_axis',(0.,1.,0.));
#74094=DIRECTION('',(0.,0.,1.));
#74095=DIRECTION('',(0.,1.,0.));
#74096=DIRECTION('center_axis',(1.,0.,0.));
#74097=DIRECTION('ref_axis',(0.,-1.,0.));
#74098=DIRECTION('',(0.,-1.,0.));
#74099=DIRECTION('',(0.,0.,-1.));
#74100=DIRECTION('',(0.,-1.,0.));
#74101=DIRECTION('center_axis',(-1.,0.,0.));
#74102=DIRECTION('ref_axis',(0.,1.,0.));
#74103=DIRECTION('',(0.,1.,0.));
#74104=DIRECTION('',(0.,0.,1.));
#74105=DIRECTION('',(0.,1.,0.));
#74106=DIRECTION('center_axis',(0.,0.,-1.));
#74107=DIRECTION('ref_axis',(-1.,0.,0.));
#74108=DIRECTION('center_axis',(0.,0.,1.));
#74109=DIRECTION('ref_axis',(1.,0.,0.));
#74110=DIRECTION('',(-1.,0.,0.));
#74111=DIRECTION('center_axis',(0.,0.,1.));
#74112=DIRECTION('ref_axis',(1.,0.,0.));
#74113=DIRECTION('',(1.,0.,0.));
#74114=DIRECTION('center_axis',(0.,0.,-1.));
#74115=DIRECTION('ref_axis',(1.,0.,0.));
#74116=DIRECTION('center_axis',(0.,0.,1.));
#74117=DIRECTION('ref_axis',(1.,0.,0.));
#74118=DIRECTION('center_axis',(0.,0.,-1.));
#74119=DIRECTION('ref_axis',(1.,0.,0.));
#74120=DIRECTION('',(1.,0.,0.));
#74121=DIRECTION('center_axis',(0.,-1.,0.));
#74122=DIRECTION('ref_axis',(1.,0.,0.));
#74123=DIRECTION('',(1.,0.,0.));
#74124=DIRECTION('',(1.,0.,0.));
#74125=DIRECTION('',(1.,0.,0.));
#74126=DIRECTION('',(1.,0.,0.));
#74127=DIRECTION('',(1.,0.,0.));
#74128=DIRECTION('',(1.,0.,0.));
#74129=DIRECTION('',(1.,0.,0.));
#74130=DIRECTION('',(1.,0.,0.));
#74131=DIRECTION('',(1.,0.,0.));
#74132=DIRECTION('',(1.,0.,0.));
#74133=DIRECTION('',(1.,0.,0.));
#74134=DIRECTION('',(1.,0.,0.));
#74135=DIRECTION('',(1.,0.,0.));
#74136=DIRECTION('',(1.,0.,0.));
#74137=DIRECTION('',(1.,0.,0.));
#74138=DIRECTION('',(1.,0.,0.));
#74139=DIRECTION('',(0.,0.,1.));
#74140=DIRECTION('',(1.,0.,0.));
#74141=DIRECTION('',(0.,0.,1.));
#74142=DIRECTION('',(1.,0.,0.));
#74143=DIRECTION('',(1.,0.,0.));
#74144=DIRECTION('center_axis',(0.,0.,1.));
#74145=DIRECTION('ref_axis',(1.,0.,0.));
#74146=DIRECTION('center_axis',(0.,0.,1.));
#74147=DIRECTION('ref_axis',(1.,0.,0.));
#74148=DIRECTION('',(0.,0.,1.));
#74149=DIRECTION('center_axis',(0.,0.,1.));
#74150=DIRECTION('ref_axis',(1.,0.,0.));
#74151=DIRECTION('center_axis',(0.,0.,1.));
#74152=DIRECTION('ref_axis',(1.,0.,0.));
#74153=DIRECTION('',(-0.707106781186554,-8.65956056235502E-17,0.707106781186541));
#74154=DIRECTION('center_axis',(0.,0.,-1.));
#74155=DIRECTION('ref_axis',(1.,0.,0.));
#74156=DIRECTION('center_axis',(0.,0.,-1.));
#74157=DIRECTION('ref_axis',(1.,0.,0.));
#74158=DIRECTION('center_axis',(0.,0.,-1.));
#74159=DIRECTION('ref_axis',(1.,0.,0.));
#74160=DIRECTION('center_axis',(0.,0.,1.));
#74161=DIRECTION('ref_axis',(1.,0.,0.));
#74162=DIRECTION('',(-1.,0.,0.));
#74163=DIRECTION('center_axis',(0.,0.,-1.));
#74164=DIRECTION('ref_axis',(1.,0.,0.));
#74165=DIRECTION('center_axis',(0.,0.,1.));
#74166=DIRECTION('ref_axis',(1.,0.,0.));
#74167=DIRECTION('',(0.,1.,0.));
#74168=DIRECTION('center_axis',(0.,0.,1.));
#74169=DIRECTION('ref_axis',(1.,0.,0.));
#74170=DIRECTION('',(-1.,0.,0.));
#74171=DIRECTION('center_axis',(0.,0.,1.));
#74172=DIRECTION('ref_axis',(1.,0.,0.));
#74173=DIRECTION('center_axis',(0.,0.,1.));
#74174=DIRECTION('ref_axis',(1.,0.,0.));
#74175=DIRECTION('',(0.,0.,1.));
#74176=DIRECTION('center_axis',(0.,0.,1.));
#74177=DIRECTION('ref_axis',(1.,0.,0.));
#74178=DIRECTION('center_axis',(0.,0.,1.));
#74179=DIRECTION('ref_axis',(1.,0.,0.));
#74180=DIRECTION('',(-0.707106781186547,-8.65956056235493E-17,0.707106781186547));
#74181=DIRECTION('center_axis',(0.,0.,-1.));
#74182=DIRECTION('ref_axis',(1.,0.,0.));
#74183=DIRECTION('center_axis',(0.,0.,-1.));
#74184=DIRECTION('ref_axis',(1.,0.,0.));
#74185=DIRECTION('center_axis',(0.,0.,1.));
#74186=DIRECTION('ref_axis',(1.,0.,0.));
#74187=DIRECTION('',(-1.,0.,0.));
#74188=DIRECTION('center_axis',(0.,0.,1.));
#74189=DIRECTION('ref_axis',(0.,1.,0.));
#74190=DIRECTION('',(0.,-1.,0.));
#74191=DIRECTION('center_axis',(0.,0.,1.));
#74192=DIRECTION('ref_axis',(0.,1.,0.));
#74193=DIRECTION('center_axis',(0.,0.,1.));
#74194=DIRECTION('ref_axis',(0.,1.,0.));
#74195=DIRECTION('',(0.,0.,1.));
#74196=DIRECTION('',(0.,0.,1.));
#74197=DIRECTION('center_axis',(0.,1.,0.));
#74198=DIRECTION('ref_axis',(-1.,0.,0.));
#74199=DIRECTION('',(0.,0.,1.));
#74200=DIRECTION('',(-1.,0.,0.));
#74201=DIRECTION('center_axis',(0.,0.,1.));
#74202=DIRECTION('ref_axis',(1.,0.,0.));
#74203=DIRECTION('center_axis',(0.,0.,1.));
#74204=DIRECTION('ref_axis',(1.,0.,0.));
#74205=DIRECTION('',(0.,0.,1.));
#74206=DIRECTION('center_axis',(1.,0.,0.));
#74207=DIRECTION('ref_axis',(0.,1.,0.));
#74208=DIRECTION('',(0.,1.,0.));
#74209=DIRECTION('center_axis',(-1.,0.,0.));
#74210=DIRECTION('ref_axis',(0.,-1.,0.));
#74211=DIRECTION('',(0.,-1.,0.));
#74212=DIRECTION('center_axis',(0.,0.,1.));
#74213=DIRECTION('ref_axis',(1.,0.,0.));
#102123=CARTESIAN_POINT('',(0.,0.,0.));
#102124=CARTESIAN_POINT('Origin',(116.37,9.4,49.7));
#102125=CARTESIAN_POINT('',(116.37,8.6,49.7));
#102126=CARTESIAN_POINT('',(116.37,8.6,49.6));
#102127=CARTESIAN_POINT('',(116.37,8.6,49.1));
#102128=CARTESIAN_POINT('',(116.37,9.4,49.7));
#102129=CARTESIAN_POINT('',(116.37,9.8,49.7));
#102130=CARTESIAN_POINT('',(116.37,9.4,49.6));
#102131=CARTESIAN_POINT('',(116.37,9.4,49.7));
#102132=CARTESIAN_POINT('',(116.37,8.5,49.6));
#102133=CARTESIAN_POINT('Origin',(116.3,8.95,49.6));
#102134=CARTESIAN_POINT('',(116.23,8.6,49.6));
#102135=CARTESIAN_POINT('',(107.65,8.6,49.6));
#102136=CARTESIAN_POINT('',(116.23,9.4,49.6));
#102137=CARTESIAN_POINT('',(116.37,9.4,49.6));
#102138=CARTESIAN_POINT('',(116.23,9.4,49.6));
#102139=CARTESIAN_POINT('Origin',(116.23,9.4,49.7));
#102140=CARTESIAN_POINT('',(116.23,9.4,49.7));
#102141=CARTESIAN_POINT('',(113.115,9.4,49.7));
#102142=CARTESIAN_POINT('',(116.23,9.4,49.7));
#102143=CARTESIAN_POINT('Origin',(116.23,8.5,49.7));
#102144=CARTESIAN_POINT('',(116.23,8.6,49.7));
#102145=CARTESIAN_POINT('',(116.23,8.6,49.1));
#102146=CARTESIAN_POINT('',(116.23,9.35,49.7));
#102147=CARTESIAN_POINT('Origin',(114.57,9.8,49.7));
#102148=CARTESIAN_POINT('',(114.57,8.6,49.7));
#102149=CARTESIAN_POINT('',(114.57,8.6,49.6));
#102150=CARTESIAN_POINT('',(114.57,8.6,49.1));
#102151=CARTESIAN_POINT('',(114.57,9.8,49.7));
#102152=CARTESIAN_POINT('',(114.57,10.,49.7));
#102153=CARTESIAN_POINT('',(114.57,9.8,49.6));
#102154=CARTESIAN_POINT('',(114.57,9.8,49.7));
#102155=CARTESIAN_POINT('',(114.57,8.5,49.6));
#102156=CARTESIAN_POINT('Origin',(114.5,9.15,49.6));
#102157=CARTESIAN_POINT('',(114.43,8.6,49.6));
#102158=CARTESIAN_POINT('',(106.75,8.6,49.6));
#102159=CARTESIAN_POINT('',(114.43,9.8,49.6));
#102160=CARTESIAN_POINT('',(114.57,9.8,49.6));
#102161=CARTESIAN_POINT('',(114.43,9.8,49.6));
#102162=CARTESIAN_POINT('Origin',(114.43,9.8,49.7));
#102163=CARTESIAN_POINT('',(114.43,9.8,49.7));
#102164=CARTESIAN_POINT('',(112.215,9.8,49.7));
#102165=CARTESIAN_POINT('',(114.43,9.8,49.7));
#102166=CARTESIAN_POINT('Origin',(114.43,8.5,49.7));
#102167=CARTESIAN_POINT('',(114.43,8.6,49.7));
#102168=CARTESIAN_POINT('',(114.43,8.6,49.1));
#102169=CARTESIAN_POINT('',(114.43,9.35,49.7));
#102170=CARTESIAN_POINT('Origin',(112.77,9.4,49.7));
#102171=CARTESIAN_POINT('',(112.77,8.6,49.7));
#102172=CARTESIAN_POINT('',(112.77,8.6,49.6));
#102173=CARTESIAN_POINT('',(112.77,8.6,49.1));
#102174=CARTESIAN_POINT('',(112.77,9.4,49.7));
#102175=CARTESIAN_POINT('',(112.77,9.8,49.7));
#102176=CARTESIAN_POINT('',(112.77,9.4,49.6));
#102177=CARTESIAN_POINT('',(112.77,9.4,49.7));
#102178=CARTESIAN_POINT('',(112.77,8.5,49.6));
#102179=CARTESIAN_POINT('Origin',(112.7,8.95,49.6));
#102180=CARTESIAN_POINT('',(112.63,8.6,49.6));
#102181=CARTESIAN_POINT('',(105.85,8.6,49.6));
#102182=CARTESIAN_POINT('',(112.63,9.4,49.6));
#102183=CARTESIAN_POINT('',(112.77,9.4,49.6));
#102184=CARTESIAN_POINT('',(112.63,9.4,49.6));
#102185=CARTESIAN_POINT('Origin',(112.63,9.4,49.7));
#102186=CARTESIAN_POINT('',(112.63,9.4,49.7));
#102187=CARTESIAN_POINT('',(111.315,9.4,49.7));
#102188=CARTESIAN_POINT('',(112.63,9.4,49.7));
#102189=CARTESIAN_POINT('Origin',(112.63,8.5,49.7));
#102190=CARTESIAN_POINT('',(112.63,8.6,49.7));
#102191=CARTESIAN_POINT('',(112.63,8.6,49.1));
#102192=CARTESIAN_POINT('',(112.63,9.35,49.7));
#102193=CARTESIAN_POINT('Origin',(110.97,9.4,49.7));
#102194=CARTESIAN_POINT('',(110.97,8.6,49.7));
#102195=CARTESIAN_POINT('',(110.97,8.6,49.6));
#102196=CARTESIAN_POINT('',(110.97,8.6,49.1));
#102197=CARTESIAN_POINT('',(110.97,9.4,49.7));
#102198=CARTESIAN_POINT('',(110.97,9.8,49.7));
#102199=CARTESIAN_POINT('',(110.97,9.4,49.6));
#102200=CARTESIAN_POINT('',(110.97,9.4,49.7));
#102201=CARTESIAN_POINT('',(110.97,8.5,49.6));
#102202=CARTESIAN_POINT('Origin',(110.9,8.95,49.6));
#102203=CARTESIAN_POINT('',(110.83,8.6,49.6));
#102204=CARTESIAN_POINT('',(104.95,8.6,49.6));
#102205=CARTESIAN_POINT('',(110.83,9.4,49.6));
#102206=CARTESIAN_POINT('',(110.97,9.4,49.6));
#102207=CARTESIAN_POINT('',(110.83,9.4,49.6));
#102208=CARTESIAN_POINT('Origin',(110.83,9.4,49.7));
#102209=CARTESIAN_POINT('',(110.83,9.4,49.7));
#102210=CARTESIAN_POINT('',(110.415,9.4,49.7));
#102211=CARTESIAN_POINT('',(110.83,9.4,49.7));
#102212=CARTESIAN_POINT('Origin',(110.83,8.5,49.7));
#102213=CARTESIAN_POINT('',(110.83,8.6,49.7));
#102214=CARTESIAN_POINT('',(110.83,8.6,49.1));
#102215=CARTESIAN_POINT('',(110.83,9.35,49.7));
#102216=CARTESIAN_POINT('Origin',(110.07,10.2,49.7));
#102217=CARTESIAN_POINT('',(110.07,8.6,49.7));
#102218=CARTESIAN_POINT('',(110.07,8.6,49.6));
#102219=CARTESIAN_POINT('',(110.07,8.6,49.1));
#102220=CARTESIAN_POINT('',(110.07,10.2,49.7));
#102221=CARTESIAN_POINT('',(110.07,10.2,49.7));
#102222=CARTESIAN_POINT('',(110.07,10.2,49.6));
#102223=CARTESIAN_POINT('',(110.07,10.2,49.7));
#102224=CARTESIAN_POINT('',(110.07,8.5,49.6));
#102225=CARTESIAN_POINT('Origin',(110.,9.35,49.6));
#102226=CARTESIAN_POINT('',(109.93,8.6,49.6));
#102227=CARTESIAN_POINT('',(104.5,8.6,49.6));
#102228=CARTESIAN_POINT('',(109.93,10.2,49.6));
#102229=CARTESIAN_POINT('',(110.07,10.2,49.6));
#102230=CARTESIAN_POINT('',(109.93,10.2,49.6));
#102231=CARTESIAN_POINT('Origin',(109.93,10.2,49.7));
#102232=CARTESIAN_POINT('',(109.93,10.2,49.7));
#102233=CARTESIAN_POINT('',(109.965,10.2,49.7));
#102234=CARTESIAN_POINT('',(109.93,10.2,49.7));
#102235=CARTESIAN_POINT('Origin',(109.93,8.5,49.7));
#102236=CARTESIAN_POINT('',(109.93,8.6,49.7));
#102237=CARTESIAN_POINT('',(109.93,8.6,49.1));
#102238=CARTESIAN_POINT('',(109.93,9.35,49.7));
#102239=CARTESIAN_POINT('Origin',(108.27,9.4,49.7));
#102240=CARTESIAN_POINT('',(108.27,8.6,49.7));
#102241=CARTESIAN_POINT('',(108.27,8.6,49.6));
#102242=CARTESIAN_POINT('',(108.27,8.6,49.1));
#102243=CARTESIAN_POINT('',(108.27,9.4,49.7));
#102244=CARTESIAN_POINT('',(108.27,9.8,49.7));
#102245=CARTESIAN_POINT('',(108.27,9.4,49.6));
#102246=CARTESIAN_POINT('',(108.27,9.4,49.7));
#102247=CARTESIAN_POINT('',(108.27,8.5,49.6));
#102248=CARTESIAN_POINT('Origin',(108.2,8.95,49.6));
#102249=CARTESIAN_POINT('',(108.13,8.6,49.6));
#102250=CARTESIAN_POINT('',(103.6,8.6,49.6));
#102251=CARTESIAN_POINT('',(108.13,9.4,49.6));
#102252=CARTESIAN_POINT('',(108.27,9.4,49.6));
#102253=CARTESIAN_POINT('',(108.13,9.4,49.6));
#102254=CARTESIAN_POINT('Origin',(108.13,9.4,49.7));
#102255=CARTESIAN_POINT('',(108.13,9.4,49.7));
#102256=CARTESIAN_POINT('',(109.065,9.4,49.7));
#102257=CARTESIAN_POINT('',(108.13,9.4,49.7));
#102258=CARTESIAN_POINT('Origin',(108.13,8.5,49.7));
#102259=CARTESIAN_POINT('',(108.13,8.6,49.7));
#102260=CARTESIAN_POINT('',(108.13,8.6,49.1));
#102261=CARTESIAN_POINT('',(108.13,9.35,49.7));
#102262=CARTESIAN_POINT('Origin',(106.47,9.4,49.7));
#102263=CARTESIAN_POINT('',(106.47,8.6,49.7));
#102264=CARTESIAN_POINT('',(106.47,8.6,49.6));
#102265=CARTESIAN_POINT('',(106.47,8.6,49.1));
#102266=CARTESIAN_POINT('',(106.47,9.4,49.7));
#102267=CARTESIAN_POINT('',(106.47,9.8,49.7));
#102268=CARTESIAN_POINT('',(106.47,9.4,49.6));
#102269=CARTESIAN_POINT('',(106.47,9.4,49.7));
#102270=CARTESIAN_POINT('',(106.47,8.5,49.6));
#102271=CARTESIAN_POINT('Origin',(106.4,8.95,49.6));
#102272=CARTESIAN_POINT('',(106.33,8.6,49.6));
#102273=CARTESIAN_POINT('',(102.7,8.6,49.6));
#102274=CARTESIAN_POINT('',(106.33,9.4,49.6));
#102275=CARTESIAN_POINT('',(106.47,9.4,49.6));
#102276=CARTESIAN_POINT('',(106.33,9.4,49.6));
#102277=CARTESIAN_POINT('Origin',(106.33,9.4,49.7));
#102278=CARTESIAN_POINT('',(106.33,9.4,49.7));
#102279=CARTESIAN_POINT('',(108.165,9.4,49.7));
#102280=CARTESIAN_POINT('',(106.33,9.4,49.7));
#102281=CARTESIAN_POINT('Origin',(106.33,8.5,49.7));
#102282=CARTESIAN_POINT('',(106.33,8.6,49.7));
#102283=CARTESIAN_POINT('',(106.33,8.6,49.1));
#102284=CARTESIAN_POINT('',(106.33,9.35,49.7));
#102285=CARTESIAN_POINT('Origin',(104.67,9.4,49.7));
#102286=CARTESIAN_POINT('',(104.67,8.6,49.7));
#102287=CARTESIAN_POINT('',(104.67,8.6,49.6));
#102288=CARTESIAN_POINT('',(104.67,8.6,49.1));
#102289=CARTESIAN_POINT('',(104.67,9.4,49.7));
#102290=CARTESIAN_POINT('',(104.67,9.8,49.7));
#102291=CARTESIAN_POINT('',(104.67,9.4,49.6));
#102292=CARTESIAN_POINT('',(104.67,9.4,49.7));
#102293=CARTESIAN_POINT('',(104.67,8.5,49.6));
#102294=CARTESIAN_POINT('Origin',(104.6,8.95,49.6));
#102295=CARTESIAN_POINT('',(104.53,8.6,49.6));
#102296=CARTESIAN_POINT('',(101.8,8.6,49.6));
#102297=CARTESIAN_POINT('',(104.53,9.4,49.6));
#102298=CARTESIAN_POINT('',(104.67,9.4,49.6));
#102299=CARTESIAN_POINT('',(104.53,9.4,49.6));
#102300=CARTESIAN_POINT('Origin',(104.53,9.4,49.7));
#102301=CARTESIAN_POINT('',(104.53,9.4,49.7));
#102302=CARTESIAN_POINT('',(107.265,9.4,49.7));
#102303=CARTESIAN_POINT('',(104.53,9.4,49.7));
#102304=CARTESIAN_POINT('Origin',(104.53,8.5,49.7));
#102305=CARTESIAN_POINT('',(104.53,8.6,49.7));
#102306=CARTESIAN_POINT('',(104.53,8.6,49.1));
#102307=CARTESIAN_POINT('',(104.53,9.35,49.7));
#102308=CARTESIAN_POINT('Origin',(102.87,9.4,49.7));
#102309=CARTESIAN_POINT('',(102.87,8.88352744046827,49.6));
#102310=CARTESIAN_POINT('',(102.87,8.74291386665029,49.7));
#102311=CARTESIAN_POINT('Ctrl Pts',(102.87,8.88352744046827,49.6));
#102312=CARTESIAN_POINT('Ctrl Pts',(102.87,8.81502339168512,49.6474651054947));
#102313=CARTESIAN_POINT('Ctrl Pts',(102.87,8.74291386665029,49.7));
#102314=CARTESIAN_POINT('',(102.87,8.6,49.6));
#102315=CARTESIAN_POINT('',(102.87,8.5,49.6));
#102316=CARTESIAN_POINT('',(102.87,8.6,49.7));
#102317=CARTESIAN_POINT('',(102.87,8.6,49.1));
#102318=CARTESIAN_POINT('',(102.87,9.8,49.7));
#102319=CARTESIAN_POINT('Origin',(102.73,8.5,49.7));
#102320=CARTESIAN_POINT('',(102.73,8.62294578406448,49.7));
#102321=CARTESIAN_POINT('',(102.73,8.75186326612437,49.6));
#102322=CARTESIAN_POINT('Ctrl Pts',(102.73,8.62294578406448,49.7));
#102323=CARTESIAN_POINT('Ctrl Pts',(102.73,8.68905731332551,49.6478692670285));
#102324=CARTESIAN_POINT('Ctrl Pts',(102.73,8.75186326612437,49.6));
#102325=CARTESIAN_POINT('',(102.73,8.6,49.7));
#102326=CARTESIAN_POINT('',(102.73,9.35,49.7));
#102327=CARTESIAN_POINT('',(102.73,8.6,49.6));
#102328=CARTESIAN_POINT('',(102.73,8.6,49.1));
#102329=CARTESIAN_POINT('',(102.73,9.4,49.6));
#102330=CARTESIAN_POINT('Origin',(102.8,8.95,49.6));
#102331=CARTESIAN_POINT('Origin',(101.5,10.2,49.6));
#102332=CARTESIAN_POINT('',(100.9,8.6,49.6));
#102333=CARTESIAN_POINT('Origin',(103.77,9.4,49.7));
#102334=CARTESIAN_POINT('',(103.77,8.6,49.7));
#102335=CARTESIAN_POINT('',(103.77,8.6,49.6));
#102336=CARTESIAN_POINT('',(103.77,8.6,49.1));
#102337=CARTESIAN_POINT('',(103.77,9.4,49.7));
#102338=CARTESIAN_POINT('',(103.77,9.8,49.7));
#102339=CARTESIAN_POINT('',(103.77,9.4,49.6));
#102340=CARTESIAN_POINT('',(103.77,9.4,49.7));
#102341=CARTESIAN_POINT('',(103.77,8.5,49.6));
#102342=CARTESIAN_POINT('Origin',(103.7,8.95,49.6));
#102343=CARTESIAN_POINT('',(103.63,8.6,49.6));
#102344=CARTESIAN_POINT('',(101.35,8.6,49.6));
#102345=CARTESIAN_POINT('',(103.63,9.4,49.6));
#102346=CARTESIAN_POINT('',(103.77,9.4,49.6));
#102347=CARTESIAN_POINT('',(103.63,9.4,49.6));
#102348=CARTESIAN_POINT('Origin',(103.63,9.4,49.7));
#102349=CARTESIAN_POINT('',(103.63,9.4,49.7));
#102350=CARTESIAN_POINT('',(106.815,9.4,49.7));
#102351=CARTESIAN_POINT('',(103.63,9.4,49.7));
#102352=CARTESIAN_POINT('Origin',(103.63,8.5,49.7));
#102353=CARTESIAN_POINT('',(103.63,8.6,49.7));
#102354=CARTESIAN_POINT('',(103.63,8.6,49.1));
#102355=CARTESIAN_POINT('',(103.63,9.35,49.7));
#102356=CARTESIAN_POINT('Origin',(105.57,9.8,49.7));
#102357=CARTESIAN_POINT('',(105.57,8.6,49.7));
#102358=CARTESIAN_POINT('',(105.57,8.6,49.6));
#102359=CARTESIAN_POINT('',(105.57,8.6,49.1));
#102360=CARTESIAN_POINT('',(105.57,9.8,49.7));
#102361=CARTESIAN_POINT('',(105.57,10.,49.7));
#102362=CARTESIAN_POINT('',(105.57,9.8,49.6));
#102363=CARTESIAN_POINT('',(105.57,9.8,49.7));
#102364=CARTESIAN_POINT('',(105.57,8.5,49.6));
#102365=CARTESIAN_POINT('Origin',(105.5,9.15,49.6));
#102366=CARTESIAN_POINT('',(105.43,8.6,49.6));
#102367=CARTESIAN_POINT('',(102.25,8.6,49.6));
#102368=CARTESIAN_POINT('',(105.43,9.8,49.6));
#102369=CARTESIAN_POINT('',(105.57,9.8,49.6));
#102370=CARTESIAN_POINT('',(105.43,9.8,49.6));
#102371=CARTESIAN_POINT('Origin',(105.43,9.8,49.7));
#102372=CARTESIAN_POINT('',(105.43,9.8,49.7));
#102373=CARTESIAN_POINT('',(107.715,9.8,49.7));
#102374=CARTESIAN_POINT('',(105.43,9.8,49.7));
#102375=CARTESIAN_POINT('Origin',(105.43,8.5,49.7));
#102376=CARTESIAN_POINT('',(105.43,8.6,49.7));
#102377=CARTESIAN_POINT('',(105.43,8.6,49.1));
#102378=CARTESIAN_POINT('',(105.43,9.35,49.7));
#102379=CARTESIAN_POINT('Origin',(107.37,9.4,49.7));
#102380=CARTESIAN_POINT('',(107.37,8.6,49.7));
#102381=CARTESIAN_POINT('',(107.37,8.6,49.6));
#102382=CARTESIAN_POINT('',(107.37,8.6,49.1));
#102383=CARTESIAN_POINT('',(107.37,9.4,49.7));
#102384=CARTESIAN_POINT('',(107.37,9.8,49.7));
#102385=CARTESIAN_POINT('',(107.37,9.4,49.6));
#102386=CARTESIAN_POINT('',(107.37,9.4,49.7));
#102387=CARTESIAN_POINT('',(107.37,8.5,49.6));
#102388=CARTESIAN_POINT('Origin',(107.3,8.95,49.6));
#102389=CARTESIAN_POINT('',(107.23,8.6,49.6));
#102390=CARTESIAN_POINT('',(103.15,8.6,49.6));
#102391=CARTESIAN_POINT('',(107.23,9.4,49.6));
#102392=CARTESIAN_POINT('',(107.37,9.4,49.6));
#102393=CARTESIAN_POINT('',(107.23,9.4,49.6));
#102394=CARTESIAN_POINT('Origin',(107.23,9.4,49.7));
#102395=CARTESIAN_POINT('',(107.23,9.4,49.7));
#102396=CARTESIAN_POINT('',(108.615,9.4,49.7));
#102397=CARTESIAN_POINT('',(107.23,9.4,49.7));
#102398=CARTESIAN_POINT('Origin',(107.23,8.5,49.7));
#102399=CARTESIAN_POINT('',(107.23,8.6,49.7));
#102400=CARTESIAN_POINT('',(107.23,8.6,49.1));
#102401=CARTESIAN_POINT('',(107.23,9.35,49.7));
#102402=CARTESIAN_POINT('Origin',(109.17,9.4,49.7));
#102403=CARTESIAN_POINT('',(109.17,8.6,49.7));
#102404=CARTESIAN_POINT('',(109.17,8.6,49.6));
#102405=CARTESIAN_POINT('',(109.17,8.6,49.1));
#102406=CARTESIAN_POINT('',(109.17,9.4,49.7));
#102407=CARTESIAN_POINT('',(109.17,9.8,49.7));
#102408=CARTESIAN_POINT('',(109.17,9.4,49.6));
#102409=CARTESIAN_POINT('',(109.17,9.4,49.7));
#102410=CARTESIAN_POINT('',(109.17,8.5,49.6));
#102411=CARTESIAN_POINT('Origin',(109.1,8.95,49.6));
#102412=CARTESIAN_POINT('',(109.03,8.6,49.6));
#102413=CARTESIAN_POINT('',(104.05,8.6,49.6));
#102414=CARTESIAN_POINT('',(109.03,9.4,49.6));
#102415=CARTESIAN_POINT('',(109.17,9.4,49.6));
#102416=CARTESIAN_POINT('',(109.03,9.4,49.6));
#102417=CARTESIAN_POINT('Origin',(109.03,9.4,49.7));
#102418=CARTESIAN_POINT('',(109.03,9.4,49.7));
#102419=CARTESIAN_POINT('',(109.515,9.4,49.7));
#102420=CARTESIAN_POINT('',(109.03,9.4,49.7));
#102421=CARTESIAN_POINT('Origin',(109.03,8.5,49.7));
#102422=CARTESIAN_POINT('',(109.03,8.6,49.7));
#102423=CARTESIAN_POINT('',(109.03,8.6,49.1));
#102424=CARTESIAN_POINT('',(109.03,9.35,49.7));
#102425=CARTESIAN_POINT('Origin',(111.87,9.4,49.7));
#102426=CARTESIAN_POINT('',(111.87,8.6,49.7));
#102427=CARTESIAN_POINT('',(111.87,8.6,49.6));
#102428=CARTESIAN_POINT('',(111.87,8.6,49.1));
#102429=CARTESIAN_POINT('',(111.87,9.4,49.7));
#102430=CARTESIAN_POINT('',(111.87,9.8,49.7));
#102431=CARTESIAN_POINT('',(111.87,9.4,49.6));
#102432=CARTESIAN_POINT('',(111.87,9.4,49.7));
#102433=CARTESIAN_POINT('',(111.87,8.5,49.6));
#102434=CARTESIAN_POINT('Origin',(111.8,8.95,49.6));
#102435=CARTESIAN_POINT('',(111.73,8.6,49.6));
#102436=CARTESIAN_POINT('',(105.4,8.6,49.6));
#102437=CARTESIAN_POINT('',(111.73,9.4,49.6));
#102438=CARTESIAN_POINT('',(111.87,9.4,49.6));
#102439=CARTESIAN_POINT('',(111.73,9.4,49.6));
#102440=CARTESIAN_POINT('Origin',(111.73,9.4,49.7));
#102441=CARTESIAN_POINT('',(111.73,9.4,49.7));
#102442=CARTESIAN_POINT('',(110.865,9.4,49.7));
#102443=CARTESIAN_POINT('',(111.73,9.4,49.7));
#102444=CARTESIAN_POINT('Origin',(111.73,8.5,49.7));
#102445=CARTESIAN_POINT('',(111.73,8.6,49.7));
#102446=CARTESIAN_POINT('',(111.73,8.6,49.1));
#102447=CARTESIAN_POINT('',(111.73,9.35,49.7));
#102448=CARTESIAN_POINT('Origin',(113.67,9.4,49.7));
#102449=CARTESIAN_POINT('',(113.67,8.6,49.7));
#102450=CARTESIAN_POINT('',(113.67,8.6,49.6));
#102451=CARTESIAN_POINT('',(113.67,8.6,49.1));
#102452=CARTESIAN_POINT('',(113.67,9.4,49.7));
#102453=CARTESIAN_POINT('',(113.67,9.8,49.7));
#102454=CARTESIAN_POINT('',(113.67,9.4,49.6));
#102455=CARTESIAN_POINT('',(113.67,9.4,49.7));
#102456=CARTESIAN_POINT('',(113.67,8.5,49.6));
#102457=CARTESIAN_POINT('Origin',(113.6,8.95,49.6));
#102458=CARTESIAN_POINT('',(113.53,8.6,49.6));
#102459=CARTESIAN_POINT('',(106.3,8.6,49.6));
#102460=CARTESIAN_POINT('',(113.53,9.4,49.6));
#102461=CARTESIAN_POINT('',(113.67,9.4,49.6));
#102462=CARTESIAN_POINT('',(113.53,9.4,49.6));
#102463=CARTESIAN_POINT('Origin',(113.53,9.4,49.7));
#102464=CARTESIAN_POINT('',(113.53,9.4,49.7));
#102465=CARTESIAN_POINT('',(111.765,9.4,49.7));
#102466=CARTESIAN_POINT('',(113.53,9.4,49.7));
#102467=CARTESIAN_POINT('Origin',(113.53,8.5,49.7));
#102468=CARTESIAN_POINT('',(113.53,8.6,49.7));
#102469=CARTESIAN_POINT('',(113.53,8.6,49.1));
#102470=CARTESIAN_POINT('',(113.53,9.35,49.7));
#102471=CARTESIAN_POINT('Origin',(115.47,9.4,49.7));
#102472=CARTESIAN_POINT('',(115.47,8.6,49.7));
#102473=CARTESIAN_POINT('',(115.47,8.6,49.6));
#102474=CARTESIAN_POINT('',(115.47,8.6,49.1));
#102475=CARTESIAN_POINT('',(115.47,9.4,49.7));
#102476=CARTESIAN_POINT('',(115.47,9.8,49.7));
#102477=CARTESIAN_POINT('',(115.47,9.4,49.6));
#102478=CARTESIAN_POINT('',(115.47,9.4,49.7));
#102479=CARTESIAN_POINT('',(115.47,8.5,49.6));
#102480=CARTESIAN_POINT('Origin',(115.4,8.95,49.6));
#102481=CARTESIAN_POINT('',(115.33,8.6,49.6));
#102482=CARTESIAN_POINT('',(107.2,8.6,49.6));
#102483=CARTESIAN_POINT('',(115.33,9.4,49.6));
#102484=CARTESIAN_POINT('',(115.47,9.4,49.6));
#102485=CARTESIAN_POINT('',(115.33,9.4,49.6));
#102486=CARTESIAN_POINT('Origin',(115.33,9.4,49.7));
#102487=CARTESIAN_POINT('',(115.33,9.4,49.7));
#102488=CARTESIAN_POINT('',(112.665,9.4,49.7));
#102489=CARTESIAN_POINT('',(115.33,9.4,49.7));
#102490=CARTESIAN_POINT('Origin',(115.33,8.5,49.7));
#102491=CARTESIAN_POINT('',(115.33,8.6,49.7));
#102492=CARTESIAN_POINT('',(115.33,8.6,49.1));
#102493=CARTESIAN_POINT('',(115.33,9.35,49.7));
#102494=CARTESIAN_POINT('Origin',(117.27,9.4,49.7));
#102495=CARTESIAN_POINT('',(117.27,8.75186326612437,49.6));
#102496=CARTESIAN_POINT('',(117.27,8.62294578406447,49.7));
#102497=CARTESIAN_POINT('Ctrl Pts',(117.27,8.75186326612437,49.6));
#102498=CARTESIAN_POINT('Ctrl Pts',(117.27,8.68905731332593,49.6478692670281));
#102499=CARTESIAN_POINT('Ctrl Pts',(117.27,8.62294578406447,49.7));
#102500=CARTESIAN_POINT('',(117.27,8.6,49.6));
#102501=CARTESIAN_POINT('',(117.27,8.5,49.6));
#102502=CARTESIAN_POINT('',(117.27,8.6,49.7));
#102503=CARTESIAN_POINT('',(117.27,8.6,49.1));
#102504=CARTESIAN_POINT('',(117.27,9.8,49.7));
#102505=CARTESIAN_POINT('Origin',(117.13,8.5,49.7));
#102506=CARTESIAN_POINT('',(117.13,8.74291386665028,49.7));
#102507=CARTESIAN_POINT('',(117.13,8.88352744046827,49.6));
#102508=CARTESIAN_POINT('Ctrl Pts',(117.13,8.74291386665028,49.7));
#102509=CARTESIAN_POINT('Ctrl Pts',(117.13,8.81502339168516,49.6474651054946));
#102510=CARTESIAN_POINT('Ctrl Pts',(117.13,8.88352744046827,49.6));
#102511=CARTESIAN_POINT('',(117.13,8.6,49.7));
#102512=CARTESIAN_POINT('',(117.13,9.35,49.7));
#102513=CARTESIAN_POINT('',(117.13,8.6,49.6));
#102514=CARTESIAN_POINT('',(117.13,8.6,49.1));
#102515=CARTESIAN_POINT('',(117.13,9.4,49.6));
#102516=CARTESIAN_POINT('Origin',(117.2,8.95,49.6));
#102517=CARTESIAN_POINT('Origin',(118.5,10.2,49.6));
#102518=CARTESIAN_POINT('',(108.1,8.6,49.6));
#102519=CARTESIAN_POINT('Origin',(110.,10.2,49.7));
#102520=CARTESIAN_POINT('',(117.3,8.6,49.7));
#102521=CARTESIAN_POINT('',(99.,8.6,49.7));
#102522=CARTESIAN_POINT('Origin',(118.5,10.2,49.7));
#102523=CARTESIAN_POINT('Origin',(110.,10.2,49.7));
#102524=CARTESIAN_POINT('',(102.7,8.6,49.7));
#102525=CARTESIAN_POINT('Origin',(101.5,10.2,49.7));
#102526=CARTESIAN_POINT('',(99.,8.6,49.7));
#102527=CARTESIAN_POINT('Origin',(99.,8.6,48.5));
#102528=CARTESIAN_POINT('',(99.,8.6,49.7));
#102529=CARTESIAN_POINT('',(99.,8.6,49.7));
#102530=CARTESIAN_POINT('',(99.,8.6,49.7));
#102531=CARTESIAN_POINT('',(99.,8.6,49.7));
#102532=CARTESIAN_POINT('',(99.,8.6,49.7));
#102533=CARTESIAN_POINT('',(99.,8.6,49.7));
#102534=CARTESIAN_POINT('',(99.,8.6,49.7));
#102535=CARTESIAN_POINT('',(99.,8.6,49.7));
#102536=CARTESIAN_POINT('',(99.,8.6,49.7));
#102537=CARTESIAN_POINT('',(99.,8.6,49.7));
#102538=CARTESIAN_POINT('',(99.,8.6,49.7));
#102539=CARTESIAN_POINT('',(99.,8.6,49.7));
#102540=CARTESIAN_POINT('',(99.,8.6,49.7));
#102541=CARTESIAN_POINT('',(99.,8.6,49.7));
#102542=CARTESIAN_POINT('',(99.,8.6,49.7));
#102543=CARTESIAN_POINT('',(100.3,8.6,49.7));
#102544=CARTESIAN_POINT('Ctrl Pts',(102.7,8.6,49.7));
#102545=CARTESIAN_POINT('Ctrl Pts',(101.5,8.6,48.98));
#102546=CARTESIAN_POINT('Ctrl Pts',(100.3,8.6,49.7));
#102547=CARTESIAN_POINT('',(99.,8.6,49.7));
#102548=CARTESIAN_POINT('',(99.,8.6,49.7));
#102549=CARTESIAN_POINT('',(99.,8.6,48.5));
#102550=CARTESIAN_POINT('',(99.,8.6,48.5));
#102551=CARTESIAN_POINT('',(121.,8.6,48.5));
#102552=CARTESIAN_POINT('',(99.,8.6,48.5));
#102553=CARTESIAN_POINT('',(121.,8.6,49.7));
#102554=CARTESIAN_POINT('',(121.,8.6,48.5));
#102555=CARTESIAN_POINT('',(119.7,8.6,49.7));
#102556=CARTESIAN_POINT('',(99.,8.6,49.7));
#102557=CARTESIAN_POINT('Ctrl Pts',(119.7,8.6,49.7));
#102558=CARTESIAN_POINT('Ctrl Pts',(118.5,8.6,48.98));
#102559=CARTESIAN_POINT('Ctrl Pts',(117.3,8.6,49.7));
#102560=CARTESIAN_POINT('',(99.,8.6,49.7));
#102561=CARTESIAN_POINT('Origin',(118.5,10.2,48.5));
#102562=CARTESIAN_POINT('',(117.4,10.2,48.5));
#102563=CARTESIAN_POINT('Origin',(118.5,10.2,48.5));
#102564=CARTESIAN_POINT('',(117.4,10.2,48.8));
#102565=CARTESIAN_POINT('',(117.4,10.2,48.5));
#102566=CARTESIAN_POINT('Origin',(118.5,10.2,48.8));
#102567=CARTESIAN_POINT('Origin',(118.5,10.2,49.25));
#102568=CARTESIAN_POINT('',(116.5,10.2,49.7));
#102569=CARTESIAN_POINT('',(116.95,10.2,49.25));
#102570=CARTESIAN_POINT('Origin',(118.5,10.2,49.7));
#102571=CARTESIAN_POINT('',(119.7,11.8,49.7));
#102572=CARTESIAN_POINT('Origin',(118.5,10.2,49.7));
#102573=CARTESIAN_POINT('',(117.3,11.8,49.7));
#102574=CARTESIAN_POINT('Ctrl Pts',(117.3,11.8,49.7));
#102575=CARTESIAN_POINT('Ctrl Pts',(118.5,11.8,48.98));
#102576=CARTESIAN_POINT('Ctrl Pts',(119.7,11.8,49.7));
#102577=CARTESIAN_POINT('Origin',(118.5,10.2,49.7));
#102578=CARTESIAN_POINT('Origin',(110.,10.2,49.7));
#102579=CARTESIAN_POINT('',(102.7,11.8,49.7));
#102580=CARTESIAN_POINT('',(120.2,11.8,49.7));
#102581=CARTESIAN_POINT('Origin',(101.5,10.2,49.7));
#102582=CARTESIAN_POINT('Origin',(110.,10.2,49.7));
#102583=CARTESIAN_POINT('',(121.,11.,49.7));
#102584=CARTESIAN_POINT('',(121.,8.6,49.7));
#102585=CARTESIAN_POINT('',(120.2,11.8,49.7));
#102586=CARTESIAN_POINT('Origin',(120.2,11.,49.7));
#102587=CARTESIAN_POINT('',(120.2,11.8,49.7));
#102588=CARTESIAN_POINT('Origin',(101.5,10.2,48.5));
#102589=CARTESIAN_POINT('',(100.4,10.2,48.5));
#102590=CARTESIAN_POINT('Origin',(101.5,10.2,48.5));
#102591=CARTESIAN_POINT('',(100.4,10.2,48.8));
#102592=CARTESIAN_POINT('',(100.4,10.2,48.5));
#102593=CARTESIAN_POINT('Origin',(101.5,10.2,48.8));
#102594=CARTESIAN_POINT('Origin',(101.5,10.2,49.25));
#102595=CARTESIAN_POINT('',(99.5,10.2,49.7));
#102596=CARTESIAN_POINT('',(99.95,10.2,49.25));
#102597=CARTESIAN_POINT('Origin',(101.5,10.2,49.7));
#102598=CARTESIAN_POINT('',(100.3,11.8,49.7));
#102599=CARTESIAN_POINT('Ctrl Pts',(100.3,11.8,49.7));
#102600=CARTESIAN_POINT('Ctrl Pts',(101.5,11.8,48.98));
#102601=CARTESIAN_POINT('Ctrl Pts',(102.7,11.8,49.7));
#102602=CARTESIAN_POINT('Origin',(101.5,10.2,49.7));
#102603=CARTESIAN_POINT('Origin',(110.,10.2,49.7));
#102604=CARTESIAN_POINT('',(99.8,11.8,49.7));
#102605=CARTESIAN_POINT('',(120.2,11.8,49.7));
#102606=CARTESIAN_POINT('',(99.,11.,49.7));
#102607=CARTESIAN_POINT('Origin',(99.8,11.,49.7));
#102608=CARTESIAN_POINT('',(99.,11.,49.7));
#102609=CARTESIAN_POINT('Origin',(99.8,11.,48.5));
#102610=CARTESIAN_POINT('',(99.8,11.8,48.5));
#102611=CARTESIAN_POINT('',(99.,11.,48.5));
#102612=CARTESIAN_POINT('Origin',(99.8,11.,48.5));
#102613=CARTESIAN_POINT('',(99.,11.,48.5));
#102614=CARTESIAN_POINT('',(99.8,11.8,48.5));
#102615=CARTESIAN_POINT('Origin',(120.2,11.8,48.5));
#102616=CARTESIAN_POINT('',(120.2,11.8,48.5));
#102617=CARTESIAN_POINT('',(120.2,11.8,48.5));
#102618=CARTESIAN_POINT('',(120.2,11.8,48.5));
#102619=CARTESIAN_POINT('Origin',(120.2,11.,48.5));
#102620=CARTESIAN_POINT('',(121.,11.,48.5));
#102621=CARTESIAN_POINT('Origin',(120.2,11.,48.5));
#102622=CARTESIAN_POINT('',(121.,11.,48.5));
#102623=CARTESIAN_POINT('Origin',(121.,8.6,48.5));
#102624=CARTESIAN_POINT('',(121.,8.6,48.5));
#102625=CARTESIAN_POINT('Origin',(99.,11.,48.5));
#102626=CARTESIAN_POINT('',(99.,11.,48.5));
#102627=CARTESIAN_POINT('Origin',(110.,10.2,48.5));
#113955=UNCERTAINTY_MEASURE_WITH_UNIT(LENGTH_MEASURE(0.01),#113985,
'DISTANCE_ACCURACY_VALUE',
'Maximum model space distance between geometric entities at asserted c
onnectivities');
#113964=UNCERTAINTY_MEASURE_WITH_UNIT(LENGTH_MEASURE(0.01),#113985,
'DISTANCE_ACCURACY_VALUE',
'Maximum model space distance between geometric entities at asserted c
onnectivities');
#113975=(
GEOMETRIC_REPRESENTATION_CONTEXT(3)
GLOBAL_UNCERTAINTY_ASSIGNED_CONTEXT((#113955))
GLOBAL_UNIT_ASSIGNED_CONTEXT((#113985,#113987,#113988))
REPRESENTATION_CONTEXT('','3D')
);
#113984=(
GEOMETRIC_REPRESENTATION_CONTEXT(3)
GLOBAL_UNCERTAINTY_ASSIGNED_CONTEXT((#113964))
GLOBAL_UNIT_ASSIGNED_CONTEXT((#113985,#113987,#113988))
REPRESENTATION_CONTEXT('','3D')
);
#113985=(
LENGTH_UNIT()
NAMED_UNIT(*)
SI_UNIT(.MILLI.,.METRE.)
);
#113987=(
NAMED_UNIT(*)
PLANE_ANGLE_UNIT()
SI_UNIT($,.RADIAN.)
);
#113988=(
NAMED_UNIT(*)
SI_UNIT($,.STERADIAN.)
SOLID_ANGLE_UNIT()
);
#113999=SHAPE_DEFINITION_REPRESENTATION(#114018,#114061);
#114018=PRODUCT_DEFINITION_SHAPE('',$,#114081);
#114061=SHAPE_REPRESENTATION('',(#62957),#113975);
#114070=PRODUCT_DEFINITION_CONTEXT('part definition',#114129,'design');
#114081=PRODUCT_DEFINITION('2026-10-05-09-50-52-624',
'Scale Pointer - Vernier Plate',#114100,#114070);
#114100=PRODUCT_DEFINITION_FORMATION('',$,#114141);
#114129=APPLICATION_CONTEXT(
'Core Data for Automotive Mechanical Design Process');
#114130=PRODUCT_CONTEXT('part definition',#114129,'mechanical');
#114141=PRODUCT('2026-10-05-09-50-52-624',
'Scale Pointer - Vernier Plate',$,(#114130));
#114290=COLOUR_RGB('Light Blue',0.38,0.62,0.78);
#114291=FILL_AREA_STYLE_COLOUR('',#114290);
#114292=FILL_AREA_STYLE('',(#114291));
#114293=SURFACE_STYLE_FILL_AREA(#114292);
#114294=SURFACE_SIDE_STYLE('',(#114293));
#114295=SURFACE_STYLE_USAGE(.BOTH.,#114294);
#114296=PRESENTATION_STYLE_ASSIGNMENT((#114295));
ENDSEC;
END-ISO-10303-21;
